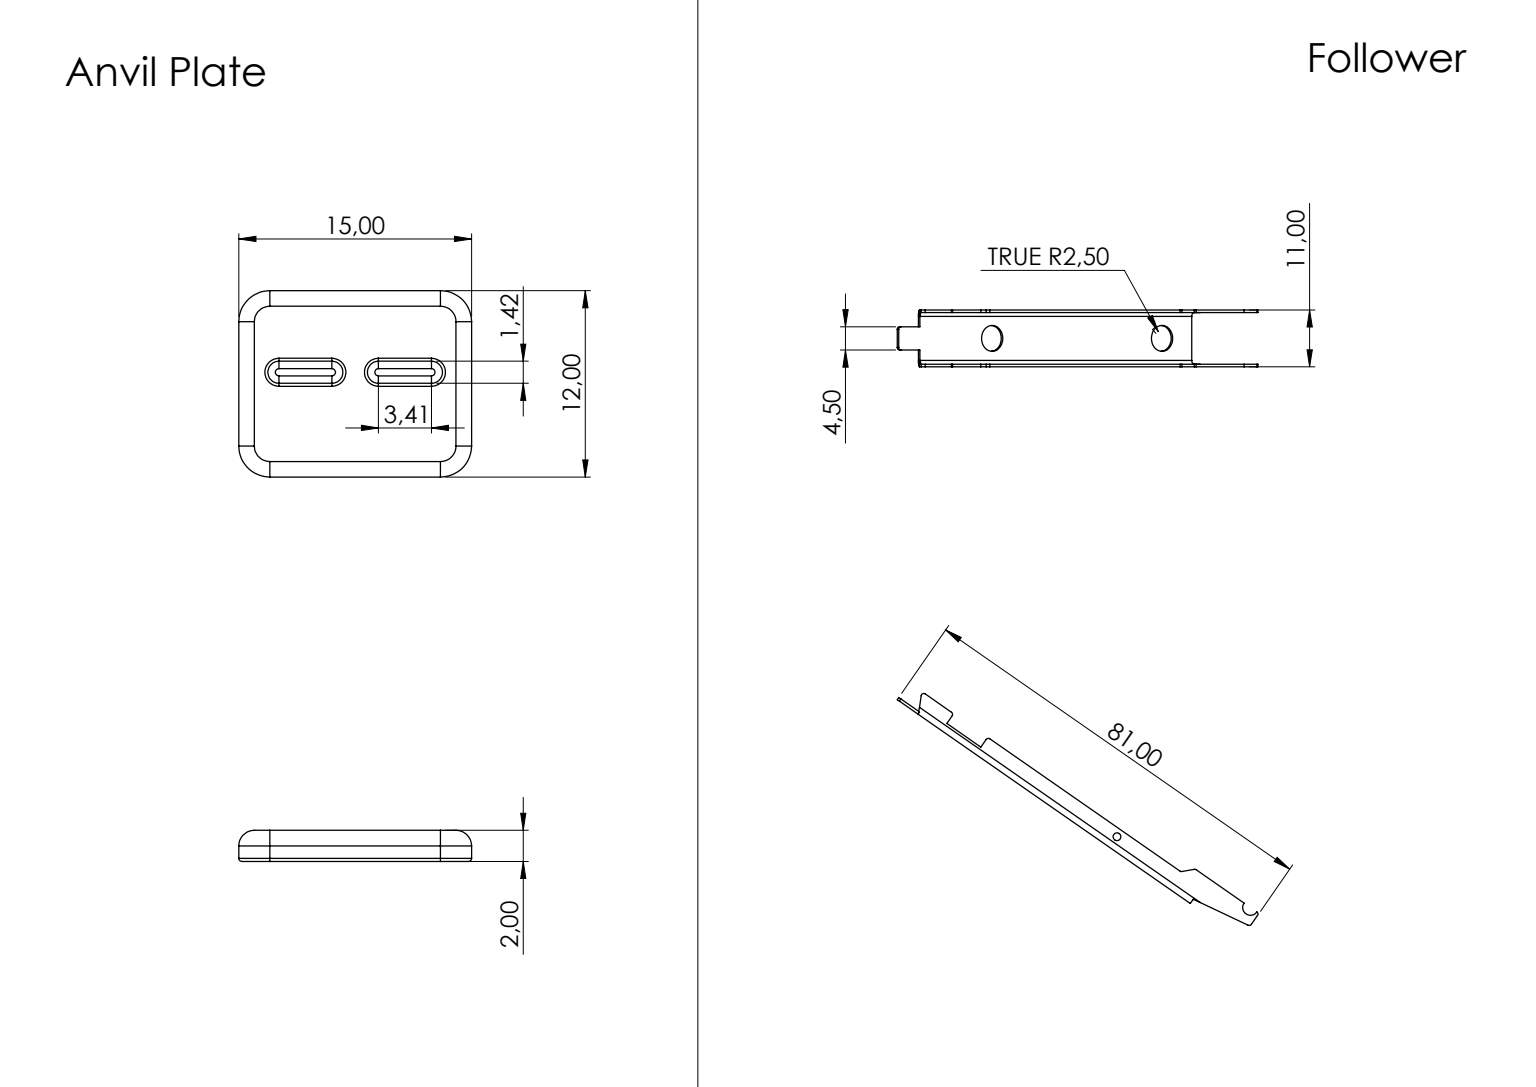
ISO-10303-21;
HEADER;
FILE_DESCRIPTION (('STEP AP214'),
    '1' );
FILE_NAME ('Follower.step',
    '2026-10-06T10:23:46',
    ( '' ),
    ( '' ),
    'SwSTEP 2.0',
    'SolidWorks 2020',
    '' );
FILE_SCHEMA (( 'AUTOMOTIVE_DESIGN' ));
ENDSEC;

DATA;
#8=FACE_OUTER_BOUND ( 'NONE', #24823, .T. ) ;
#39=B_SPLINE_SURFACE_WITH_KNOTS ( 'NONE', 1, 3, ( 
 ( #3682, #6010, #7951, #7688 ),
 ( #11564, #15795, #4076, #7569 ) ),
 .UNSPECIFIED., .F., .F., .F.,
 ( 2, 2 ),
 ( 4, 4 ),
 ( 0.000000000000000000, 1.000000000000000000 ),
 ( 0.000000000000000000, 1.000000000000000000 ),
 .UNSPECIFIED. ) ;
#42=ORIENTED_EDGE ( 'NONE', *, *, #4052, .T. ) ;
#43=CARTESIAN_POINT ( 'NONE',  ( 33.24020206407681144, 3.104049617356281932, 6.135536031321588091 ) ) ;
#48=AXIS2_PLACEMENT_3D ( 'NONE', #18248, #195, #19789 ) ;
#56=ORIENTED_EDGE ( 'NONE', *, *, #3919, .F. ) ;
#59=VERTEX_POINT ( 'NONE', #24601 ) ;
#81=CARTESIAN_POINT ( 'NONE',  ( 43.81606138205700063, -33.39268736607245103, 60.15578379404454523 ) ) ;
#87=VECTOR ( 'NONE', #691, 1000.000000000000114 ) ;
#100=DIRECTION ( 'NONE',  ( 0.000000000000000000, -0.5706330172266907974, 0.8212051873014217795 ) ) ;
#109=EDGE_CURVE ( 'NONE', #2100, #16742, #24351, .T. ) ;
#130=FACE_OUTER_BOUND ( 'NONE', #3742, .T. ) ;
#134=DIRECTION ( 'NONE',  ( 0.000000000000000000, -0.8212051873014223347, -0.5706330172266899092 ) ) ;
#140=CARTESIAN_POINT ( 'NONE',  ( 33.63257508155574271, 2.837830513113388076, 6.099065269017614810 ) ) ;
#156=ORIENTED_EDGE ( 'NONE', *, *, #18156, .F. ) ;
#170=VERTEX_POINT ( 'NONE', #12668 ) ;
#182=CARTESIAN_POINT ( 'NONE',  ( 42.90896497783001706, 3.030042170879425178, 6.235548050178295831 ) ) ;
#195=DIRECTION ( 'NONE',  ( 1.000000000000000000, -0.000000000000000000, 0.000000000000000000 ) ) ;
#198=EDGE_CURVE ( 'NONE', #24709, #13605, #5816, .T. ) ;
#199=EDGE_CURVE ( 'NONE', #8460, #24765, #19336, .T. ) ;
#205=LINE ( 'NONE', #24148, #14945 ) ;
#230=DIRECTION ( 'NONE',  ( 1.000000000000000000, 1.518641380243644581E-16, 1.055262346480601087E-16 ) ) ;
#232=CARTESIAN_POINT ( 'NONE',  ( 32.81606138205700773, -27.11289203277224402, 56.96090842897168471 ) ) ;
#233=DIRECTION ( 'NONE',  ( -1.849283715844614702E-16, 0.8212051873014210024, 0.5706330172266920187 ) ) ;
#252=ADVANCED_FACE ( 'NONE', ( #23316 ), #17669, .F. ) ;
#281=DIRECTION ( 'NONE',  ( 1.000000000000000000, 1.187136597504755470E-16, 8.249087426255173666E-17 ) ) ;
#295=B_SPLINE_CURVE_WITH_KNOTS ( 'NONE', 3,
 ( #12547, #1271, #23035, #14456, #20383, #15309, #9152 ),
 .UNSPECIFIED., .F., .F.,
 ( 4, 3, 4 ),
 ( 0.000000000000000000, 0.9999934796777874002, 1.000000000000000000 ),
 .UNSPECIFIED. ) ;
#300=DIRECTION ( 'NONE',  ( 0.000000000000000000, -0.8212051873014210024, -0.5706330172266920187 ) ) ;
#303=ORIENTED_EDGE ( 'NONE', *, *, #10224, .F. ) ;
#326=CARTESIAN_POINT ( 'NONE',  ( 42.82259893474252266, 3.224890024296139135, 6.370941811568299862 ) ) ;
#340=CARTESIAN_POINT ( 'NONE',  ( 35.81606138205700063, -6.549308025893449070, 20.35783565644092619 ) ) ;
#350=CARTESIAN_POINT ( 'NONE',  ( 42.98956905832248765, 3.335839619497401376, 6.349669990345183201 ) ) ;
#354=DIRECTION ( 'NONE',  ( -0.6683808861234329379, -0.6108281792586462977, -0.4244477900618892630 ) ) ;
#366=VECTOR ( 'NONE', #18918, 1000.000000000000114 ) ;
#374=CYLINDRICAL_SURFACE ( 'NONE', #2185, 1.500000000000006217 ) ;
#377=DIRECTION ( 'NONE',  ( 0.000000000000000000, 0.8212051873014208914, 0.5706330172266919076 ) ) ;
#406=ORIENTED_EDGE ( 'NONE', *, *, #18732, .F. ) ;
#420=ADVANCED_FACE ( 'NONE', ( #130 ), #10070, .F. ) ;
#422=EDGE_CURVE ( 'NONE', #6624, #2302, #15968, .T. ) ;
#435=ORIENTED_EDGE ( 'NONE', *, *, #25058, .T. ) ;
#455=ORIENTED_EDGE ( 'NONE', *, *, #16653, .F. ) ;
#468=EDGE_LOOP ( 'NONE', ( #17209, #1468 ) ) ;
#469=DIRECTION ( 'NONE',  ( 1.444147469618246167E-16, -0.8212051873014210024, -0.5706330172266920187 ) ) ;
#494=ORIENTED_EDGE ( 'NONE', *, *, #8342, .T. ) ;
#513=AXIS2_PLACEMENT_3D ( 'NONE', #8102, #24168, #14160 ) ;
#514=CARTESIAN_POINT ( 'NONE',  ( 33.31606138205700773, -20.26871824316192061, 44.92082169825412308 ) ) ;
#530=EDGE_LOOP ( 'NONE', ( #17922, #3533, #2092, #3855 ) ) ;
#538=PLANE ( 'NONE',  #4659 ) ;
#543=AXIS2_PLACEMENT_3D ( 'NONE', #16608, #5020, #14671 ) ;
#554=EDGE_CURVE ( 'NONE', #25393, #22104, #18436, .T. ) ;
#556=DIRECTION ( 'NONE',  ( 0.000000000000000000, -0.8212051873014223347, -0.5706330172266899092 ) ) ;
#564=CARTESIAN_POINT ( 'NONE',  ( 36.06606138205700063, 3.151453266960317023, 6.397347472316774031 ) ) ;
#592=DIRECTION ( 'NONE',  ( 0.000000000000000000, -0.5706330172266919076, 0.8212051873014208914 ) ) ;
#601=CARTESIAN_POINT ( 'NONE',  ( 32.81606138205700773, 6.705285648480822758, 7.416521610403067122 ) ) ;
#630=CARTESIAN_POINT ( 'NONE',  ( 32.81606138205700773, -35.82531359714782582, 71.25150419970752580 ) ) ;
#633=DIRECTION ( 'NONE',  ( 1.445602896647339656E-16, -0.8212051873014208914, -0.5706330172266919076 ) ) ;
#638=LINE ( 'NONE', #8521, #20462 ) ;
#644=CARTESIAN_POINT ( 'NONE',  ( 33.57054761034910229, 3.412271088041349820, 6.349711998884802533 ) ) ;
#681=ORIENTED_EDGE ( 'NONE', *, *, #198, .T. ) ;
#682=ORIENTED_EDGE ( 'NONE', *, *, #24180, .T. ) ;
#689=ORIENTED_EDGE ( 'NONE', *, *, #21380, .T. ) ;
#691=DIRECTION ( 'NONE',  ( 0.000000000000000000, -0.5706330172266919076, 0.8212051873014208914 ) ) ;
#696=AXIS2_PLACEMENT_3D ( 'NONE', #4403, #12150, #17812 ) ;
#699=EDGE_CURVE ( 'NONE', #20637, #17728, #13096, .T. ) ;
#702=ORIENTED_EDGE ( 'NONE', *, *, #17759, .F. ) ;
#713=CIRCLE ( 'NONE', #8125, 2.500000000000002220 ) ;
#769=VECTOR ( 'NONE', #7198, 1000.000000000000114 ) ;
#788=B_SPLINE_CURVE_WITH_KNOTS ( 'NONE', 3,
 ( #10750, #931, #8822, #10874 ),
 .UNSPECIFIED., .F., .F.,
 ( 4, 4 ),
 ( 0.000000000000000000, 1.000000000000000000 ),
 .UNSPECIFIED. ) ;
#792=CARTESIAN_POINT ( 'NONE',  ( 33.31606138205700773, -27.17722769842920272, 59.42551550655435477 ) ) ;
#794=LINE ( 'NONE', #9887, #17878 ) ;
#798=ORIENTED_EDGE ( 'NONE', *, *, #889, .T. ) ;
#801=DIRECTION ( 'NONE',  ( 1.444147469618246167E-16, -0.8212051873014210024, -0.5706330172266920187 ) ) ;
#814=ORIENTED_EDGE ( 'NONE', *, *, #2858, .T. ) ;
#816=CARTESIAN_POINT ( 'NONE',  ( 42.99361969242278292, 2.839052459004266726, 6.102834979010582472 ) ) ;
#818=VECTOR ( 'NONE', #17657, 1000.000000000000114 ) ;
#833=DIRECTION ( 'NONE',  ( 0.000000000000000000, -0.8212051873014208914, -0.5706330172266919076 ) ) ;
#839=EDGE_CURVE ( 'NONE', #20815, #9471, #19260, .T. ) ;
#853=LINE ( 'NONE', #22510, #16556 ) ;
#855=DIRECTION ( 'NONE',  ( 1.000000000000000000, -0.000000000000000000, 0.000000000000000000 ) ) ;
#860=CYLINDRICAL_SURFACE ( 'NONE', #7319, 0.4999999999999998890 ) ;
#861=B_SPLINE_CURVE_WITH_KNOTS ( 'NONE', 3,
 ( #25078, #7720, #7463, #19426 ),
 .UNSPECIFIED., .F., .F.,
 ( 4, 4 ),
 ( 0.000000000000000000, 1.000000000000000000 ),
 .UNSPECIFIED. ) ;
#864=ORIENTED_EDGE ( 'NONE', *, *, #11208, .F. ) ;
#872=DIRECTION ( 'NONE',  ( 1.000000000000000000, -0.000000000000000000, 0.000000000000000000 ) ) ;
#887=AXIS2_PLACEMENT_3D ( 'NONE', #14310, #8262, #20232 ) ;
#889=EDGE_CURVE ( 'NONE', #2214, #17745, #3160, .T. ) ;
#892=CARTESIAN_POINT ( 'NONE',  ( 43.81606138205700063, -27.52349462642295208, 56.67559192035834315 ) ) ;
#897=CARTESIAN_POINT ( 'NONE',  ( 33.31606138205700773, -2.088476903695762665, 19.19551655256602984 ) ) ;
#922=VECTOR ( 'NONE', #13989, 1000.000000000000114 ) ;
#926=DIRECTION ( 'NONE',  ( 0.000000000000000000, 0.8212051873014208914, 0.5706330172266919076 ) ) ;
#931=CARTESIAN_POINT ( 'NONE',  ( 33.56669025312649524, 3.416671603466172602, 6.349359658337577983 ) ) ;
#933=AXIS2_PLACEMENT_3D ( 'NONE', #16052, #8463, #9892 ) ;
#952=VERTEX_POINT ( 'NONE', #19387 ) ;
#960=ORIENTED_EDGE ( 'NONE', *, *, #16869, .T. ) ;
#965=FACE_OUTER_BOUND ( 'NONE', #17968, .T. ) ;
#967=CIRCLE ( 'NONE', #4280, 0.4999999999999994449 ) ;
#998=CARTESIAN_POINT ( 'NONE',  ( 43.06468080341912241, 3.415100481987971115, 6.350457055188933886 ) ) ;
#999=FACE_OUTER_BOUND ( 'NONE', #16254, .T. ) ;
#1002=VERTEX_POINT ( 'NONE', #21585 ) ;
#1004=CARTESIAN_POINT ( 'NONE',  ( 32.81606138205700773, -27.11289203277224402, 56.96090842897168471 ) ) ;
#1005=ORIENTED_EDGE ( 'NONE', *, *, #20302, .F. ) ;
#1025=FACE_OUTER_BOUND ( 'NONE', #16753, .T. ) ;
#1040=EDGE_CURVE ( 'NONE', #24026, #19555, #16326, .T. ) ;
#1042=EDGE_CURVE ( 'NONE', #9104, #4853, #5608, .T. ) ;
#1044=DIRECTION ( 'NONE',  ( 1.000000000000000000, -0.000000000000000000, 0.000000000000000000 ) ) ;
#1067=ORIENTED_EDGE ( 'NONE', *, *, #19250, .F. ) ;
#1068=DIRECTION ( 'NONE',  ( 1.000000000000000000, -0.000000000000000000, 0.000000000000000000 ) ) ;
#1080=LINE ( 'NONE', #15257, #5531 ) ;
#1082=FACE_OUTER_BOUND ( 'NONE', #2152, .T. ) ;
#1090=CARTESIAN_POINT ( 'NONE',  ( 42.56606138205700063, -32.75315594507191008, 59.38245422252773409 ) ) ;
#1100=CARTESIAN_POINT ( 'NONE',  ( 43.39709375099405975, 3.108381023609500193, 6.137326095127844994 ) ) ;
#1101=CARTESIAN_POINT ( 'NONE',  ( 33.31606138205700773, -26.01295748837380373, 65.89261741282676610 ) ) ;
#1103=AXIS2_PLACEMENT_3D ( 'NONE', #24593, #16498, #10723 ) ;
#1120=CIRCLE ( 'NONE', #696, 0.4999999999999982792 ) ;
#1124=EDGE_CURVE ( 'NONE', #13033, #3938, #8531, .T. ) ;
#1136=AXIS2_PLACEMENT_3D ( 'NONE', #5636, #11329, #11196 ) ;
#1146=LINE ( 'NONE', #22672, #19035 ) ;
#1159=CARTESIAN_POINT ( 'NONE',  ( 32.81606138205700773, -20.26871824316192061, 44.92082169825412308 ) ) ;
#1165=CARTESIAN_POINT ( 'NONE',  ( 32.81606138205700773, -3.566646240838321269, 18.16837712155798457 ) ) ;
#1169=ORIENTED_EDGE ( 'NONE', *, *, #18390, .F. ) ;
#1176=DIRECTION ( 'NONE',  ( -1.000000000000000000, 4.152573584826051666E-20, -5.976021130153593973E-20 ) ) ;
#1182=ORIENTED_EDGE ( 'NONE', *, *, #7364, .T. ) ;
#1191=LINE ( 'NONE', #21171, #9841 ) ;
#1194=CARTESIAN_POINT ( 'NONE',  ( 43.81608638205700146, -3.566646240838321269, 18.16837712155798457 ) ) ;
#1200=CARTESIAN_POINT ( 'NONE',  ( 32.81606138205700773, -27.60498114914039647, 57.04949906928990089 ) ) ;
#1203=VECTOR ( 'NONE', #13238, 999.9999999999998863 ) ;
#1207=CARTESIAN_POINT ( 'NONE',  ( 43.24580177837434292, 3.721690752961224202, 6.335617458560805382 ) ) ;
#1212=LINE ( 'NONE', #10894, #2646 ) ;
#1240=DIRECTION ( 'NONE',  ( 1.000000000000000000, -0.000000000000000000, 0.000000000000000000 ) ) ;
#1262=CARTESIAN_POINT ( 'NONE',  ( 33.31606138205700773, 6.366250835946937414, 6.636353555660924997 ) ) ;
#1271=CARTESIAN_POINT ( 'NONE',  ( 42.65336712727322777, 3.163553052512885877, 6.379934517999310550 ) ) ;
#1304=ORIENTED_EDGE ( 'NONE', *, *, #10169, .T. ) ;
#1316=EDGE_CURVE ( 'NONE', #2214, #22818, #6046, .T. ) ;
#1321=DIRECTION ( 'NONE',  ( 0.000000000000000000, 0.5706330172266920187, -0.8212051873014210024 ) ) ;
#1332=CARTESIAN_POINT ( 'NONE',  ( 33.23377616717382921, 3.110315666471061391, 6.136481299340784012 ) ) ;
#1348=CARTESIAN_POINT ( 'NONE',  ( 32.81606138205700773, -1.677874310045055051, 19.48083306117937852 ) ) ;
#1371=AXIS2_PLACEMENT_3D ( 'NONE', #16139, #21574, #22069 ) ;
#1372=ORIENTED_EDGE ( 'NONE', *, *, #7692, .T. ) ;
#1377=ADVANCED_FACE ( 'NONE', ( #1082 ), #8967, .T. ) ;
#1392=CARTESIAN_POINT ( 'NONE',  ( 43.31606138205700063, 6.355893005198818280, 6.643287643123708008 ) ) ;
#1412=LINE ( 'NONE', #8779, #21644 ) ;
#1433=DIRECTION ( 'NONE',  ( -1.000000000000000000, 0.000000000000000000, 0.000000000000000000 ) ) ;
#1447=VECTOR ( 'NONE', #3335, 1000.000000000000114 ) ;
#1449=DIRECTION ( 'NONE',  ( 0.000000000000000000, 0.8212051873014208914, 0.5706330172266919076 ) ) ;
#1459=ORIENTED_EDGE ( 'NONE', *, *, #3158, .F. ) ;
#1467=CARTESIAN_POINT ( 'NONE',  ( 43.70349364522802205, 3.546438648963166962, 6.213839566231161626 ) ) ;
#1468=ORIENTED_EDGE ( 'NONE', *, *, #8169, .T. ) ;
#1472=CARTESIAN_POINT ( 'NONE',  ( 32.81606138205700773, -21.50052602411404834, 44.06487217241408416 ) ) ;
#1477=CARTESIAN_POINT ( 'NONE',  ( 43.81606138205700063, -27.11289203277224402, 56.96090842897168471 ) ) ;
#1480=CARTESIAN_POINT ( 'NONE',  ( 43.79080625344859357, -32.95845724189726411, 59.23979596822106686 ) ) ;
#1491=ADVANCED_FACE ( 'NONE', ( #15640 ), #17326, .F. ) ;
#1495=CARTESIAN_POINT ( 'NONE',  ( 42.56606138205700063, 3.151453266960317023, 6.397347472316774031 ) ) ;
#1509=CARTESIAN_POINT ( 'NONE',  ( 43.38751061443460344, 3.099069811988895751, 6.135932541694130826 ) ) ;
#1510=VERTEX_POINT ( 'NONE', #1472 ) ;
#1523=CARTESIAN_POINT ( 'NONE',  ( 33.71979045277213061, 3.032422752665409060, 6.234282092415138976 ) ) ;
#1525=ADVANCED_FACE ( 'NONE', ( #3920 ), #7918, .F. ) ;
#1526=CARTESIAN_POINT ( 'NONE',  ( 43.79080625344859357, -32.95845724189726411, 59.23979596822106686 ) ) ;
#1537=VERTEX_POINT ( 'NONE', #25024 ) ;
#1543=ORIENTED_EDGE ( 'NONE', *, *, #2231, .T. ) ;
#1547=ORIENTED_EDGE ( 'NONE', *, *, #2650, .T. ) ;
#1559=AXIS2_PLACEMENT_3D ( 'NONE', #18264, #6280, #592 ) ;
#1585=DIRECTION ( 'NONE',  ( 1.000000000000000000, -0.000000000000000000, 0.000000000000000000 ) ) ;
#1588=VECTOR ( 'NONE', #24821, 1000.000000000000000 ) ;
#1595=CIRCLE ( 'NONE', #11502, 0.4999999999999943379 ) ;
#1603=ORIENTED_EDGE ( 'NONE', *, *, #4465, .F. ) ;
#1614=ORIENTED_EDGE ( 'NONE', *, *, #11768, .T. ) ;
#1617=CARTESIAN_POINT ( 'NONE',  ( 42.99670445188912282, 2.835726111602991040, 6.100265081570795722 ) ) ;
#1626=FACE_OUTER_BOUND ( 'NONE', #15605, .T. ) ;
#1628=CARTESIAN_POINT ( 'NONE',  ( 43.81606138205700063, -2.088476903695762665, 19.19551655256602984 ) ) ;
#1643=AXIS2_PLACEMENT_3D ( 'NONE', #20107, #18312, #377 ) ;
#1648=VECTOR ( 'NONE', #872, 1000.000000000000000 ) ;
#1657=LINE ( 'NONE', #23301, #818 ) ;
#1658=VERTEX_POINT ( 'NONE', #2351 ) ;
#1677=LINE ( 'NONE', #21275, #16046 ) ;
#1680=CARTESIAN_POINT ( 'NONE',  ( 33.91846891627784544, 2.749301080711977985, 6.091107676698986673 ) ) ;
#1682=DIRECTION ( 'NONE',  ( 0.000000000000000000, 0.8212051873014208914, 0.5706330172266919076 ) ) ;
#1683=EDGE_CURVE ( 'NONE', #18636, #16606, #16266, .T. ) ;
#1687=DIRECTION ( 'NONE',  ( 0.000000000000000000, 0.5706330172266920187, -0.8212051873014210024 ) ) ;
#1735=ORIENTED_EDGE ( 'NONE', *, *, #22580, .T. ) ;
#1746=ORIENTED_EDGE ( 'NONE', *, *, #21067, .T. ) ;
#1750=DIRECTION ( 'NONE',  ( -1.000000000000000000, -4.949452455753099023E-16, 7.122819585028524934E-16 ) ) ;
#1752=DIRECTION ( 'NONE',  ( 0.000000000000000000, -0.5706330172266907974, 0.8212051873014217795 ) ) ;
#1783=CARTESIAN_POINT ( 'NONE',  ( 35.81606138205700063, -29.78523130861184498, 52.92072663988442116 ) ) ;
#1801=DIRECTION ( 'NONE',  ( -1.000000000000000000, 0.000000000000000000, 0.000000000000000000 ) ) ;
#1816=DIRECTION ( 'NONE',  ( -1.000000000000000000, 0.000000000000000000, 0.000000000000000000 ) ) ;
#1847=ORIENTED_EDGE ( 'NONE', *, *, #19132, .T. ) ;
#1855=CARTESIAN_POINT ( 'NONE',  ( 43.80758610329830560, -33.17626767724734549, 59.69730752409159180 ) ) ;
#1860=ORIENTED_EDGE ( 'NONE', *, *, #12473, .T. ) ;
#1861=CARTESIAN_POINT ( 'NONE',  ( 43.81606138205700063, 6.699978067258562042, 7.424159817622362212 ) ) ;
#1882=DIRECTION ( 'NONE',  ( 0.000000000000000000, -0.5706330172266919076, 0.8212051873014208914 ) ) ;
#1890=ORIENTED_EDGE ( 'NONE', *, *, #8714, .T. ) ;
#1893=ORIENTED_EDGE ( 'NONE', *, *, #12474, .F. ) ;
#1898=CARTESIAN_POINT ( 'NONE',  ( 36.06606138205700063, 5.308699250829721272, 2.416607620847027960 ) ) ;
#1929=VECTOR ( 'NONE', #6753, 1000.000000000000114 ) ;
#1938=CARTESIAN_POINT ( 'NONE',  ( 34.06606138205700773, 2.736744647373095418, 6.109177798617293931 ) ) ;
#1946=AXIS2_PLACEMENT_3D ( 'NONE', #15039, #5257, #19545 ) ;
#1955=CARTESIAN_POINT ( 'NONE',  ( 40.06606138205700063, 5.594015759443068170, 2.006005027196319901 ) ) ;
#1964=AXIS2_PLACEMENT_3D ( 'NONE', #22242, #18267, #23913 ) ;
#1967=SURFACE_STYLE_USAGE ( .BOTH. , #7915 ) ;
#1973=LINE ( 'NONE', #9856, #22899 ) ;
#2000=AXIS2_PLACEMENT_3D ( 'NONE', #9286, #12766, #22537 ) ;
#2007=ORIENTED_EDGE ( 'NONE', *, *, #17291, .T. ) ;
#2021=AXIS2_PLACEMENT_3D ( 'NONE', #13128, #4749, #12753 ) ;
#2025=ORIENTED_EDGE ( 'NONE', *, *, #18387, .T. ) ;
#2026=VERTEX_POINT ( 'NONE', #3621 ) ;
#2039=CARTESIAN_POINT ( 'NONE',  ( 33.31606138205700773, -33.70281195181703993, 69.07320514641659770 ) ) ;
#2053=ORIENTED_EDGE ( 'NONE', *, *, #3718, .F. ) ;
#2060=PLANE ( 'NONE',  #11156 ) ;
#2064=CARTESIAN_POINT ( 'NONE',  ( 40.56606138205700773, 3.151453266960317023, 6.397347472316774031 ) ) ;
#2069=FACE_OUTER_BOUND ( 'NONE', #20298, .T. ) ;
#2070=VECTOR ( 'NONE', #18574, 1000.000000000000000 ) ;
#2092=ORIENTED_EDGE ( 'NONE', *, *, #11384, .F. ) ;
#2100=VERTEX_POINT ( 'NONE', #21035 ) ;
#2110=DIRECTION ( 'NONE',  ( 0.000000000000000000, -0.5706330172266913525, 0.8212051873014213355 ) ) ;
#2118=DIRECTION ( 'NONE',  ( -1.000000000000000000, 0.000000000000000000, 0.000000000000000000 ) ) ;
#2134=VERTEX_POINT ( 'NONE', #17170 ) ;
#2136=DIRECTION ( 'NONE',  ( 0.000000000000000000, -0.5706330172266919076, 0.8212051873014208914 ) ) ;
#2138=LINE ( 'NONE', #18006, #20063 ) ;
#2139=DIRECTION ( 'NONE',  ( -1.000000000000000000, -1.187136597504755470E-16, -8.249087426255173666E-17 ) ) ;
#2151=EDGE_CURVE ( 'NONE', #23532, #22006, #19727, .T. ) ;
#2152=EDGE_LOOP ( 'NONE', ( #3581, #6754, #7192, #10219 ) ) ;
#2157=VECTOR ( 'NONE', #20748, 1000.000000000000000 ) ;
#2163=ADVANCED_FACE ( 'NONE', ( #19632 ), #15390, .F. ) ;
#2166=CARTESIAN_POINT ( 'NONE',  ( 42.99362197529018914, 2.839053354292388143, 6.102835146812753742 ) ) ;
#2168=VECTOR ( 'NONE', #22569, 1000.000000000000114 ) ;
#2174=CARTESIAN_POINT ( 'NONE',  ( 38.31606138205700063, -29.78523130861184143, 52.92072663988442116 ) ) ;
#2185=AXIS2_PLACEMENT_3D ( 'NONE', #8014, #22033, #15852 ) ;
#2193=DIRECTION ( 'NONE',  ( -1.000000000000000000, 0.000000000000000000, 0.000000000000000000 ) ) ;
#2206=B_SPLINE_CURVE_WITH_KNOTS ( 'NONE', 3,
 ( #8105, #15951, #2539, #6429, #4246, #10424 ),
 .UNSPECIFIED., .F., .F.,
 ( 4, 2, 4 ),
 ( 0.000000000000000000, 0.5000000000000000000, 1.000000000000000000 ),
 .UNSPECIFIED. ) ;
#2207=CARTESIAN_POINT ( 'NONE',  ( 43.21596744901363962, 3.650325757544471195, 6.335220020744675828 ) ) ;
#2214=VERTEX_POINT ( 'NONE', #13842 ) ;
#2225=AXIS2_PLACEMENT_3D ( 'NONE', #3016, #16941, #7154 ) ;
#2231=EDGE_CURVE ( 'NONE', #3938, #16606, #1973, .T. ) ;
#2244=DIRECTION ( 'NONE',  ( 0.6571615412467028960, -0.6189832172005511612, -0.4301145028132777881 ) ) ;
#2259=DIRECTION ( 'NONE',  ( -1.000000000000000000, 0.000000000000000000, 0.000000000000000000 ) ) ;
#2267=CARTESIAN_POINT ( 'NONE',  ( 32.81606138205700773, 2.740850673309605412, 6.112030963703427133 ) ) ;
#2271=AXIS2_PLACEMENT_3D ( 'NONE', #630, #4518, #19980 ) ;
#2295=LINE ( 'NONE', #5926, #23610 ) ;
#2302=VERTEX_POINT ( 'NONE', #23240 ) ;
#2322=EDGE_CURVE ( 'NONE', #6643, #22414, #10576, .T. ) ;
#2335=VECTOR ( 'NONE', #4912, 1000.000000000000114 ) ;
#2351=CARTESIAN_POINT ( 'NONE',  ( 43.81606138205700063, 0.9984178969752143251, 11.59873562314662010 ) ) ;
#2353=VERTEX_POINT ( 'NONE', #10618 ) ;
#2355=CARTESIAN_POINT ( 'NONE',  ( 33.63430211860926278, 2.841683824787794688, 6.101742829876990015 ) ) ;
#2369=AXIS2_PLACEMENT_3D ( 'NONE', #14550, #4758, #9023 ) ;
#2375=VECTOR ( 'NONE', #15926, 1000.000000000000000 ) ;
#2377=ORIENTED_EDGE ( 'NONE', *, *, #11194, .F. ) ;
#2387=ORIENTED_EDGE ( 'NONE', *, *, #23881, .F. ) ;
#2389=ORIENTED_EDGE ( 'NONE', *, *, #12473, .F. ) ;
#2402=EDGE_LOOP ( 'NONE', ( #20983, #1543, #25185, #10638 ) ) ;
#2421=LINE ( 'NONE', #8239, #8598 ) ;
#2459=EDGE_LOOP ( 'NONE', ( #2389, #9279, #960, #1890 ) ) ;
#2493=ORIENTED_EDGE ( 'NONE', *, *, #20622, .F. ) ;
#2498=CARTESIAN_POINT ( 'NONE',  ( 43.31606138205700063, 6.699978067258562042, 7.424159817622362212 ) ) ;
#2504=LINE ( 'NONE', #16287, #25087 ) ;
#2505=CARTESIAN_POINT ( 'NONE',  ( 36.06606138205700063, 6.004618353093779781, 2.291321535809666354 ) ) ;
#2507=CARTESIAN_POINT ( 'NONE',  ( 40.06606138205700063, 5.719301844480432884, 2.701924129460374413 ) ) ;
#2519=PLANE ( 'NONE',  #1559 ) ;
#2536=PLANE ( 'NONE',  #20690 ) ;
#2539=CARTESIAN_POINT ( 'NONE',  ( 32.85323118609061055, 3.754743573466610140, 6.231177976620426051 ) ) ;
#2544=ADVANCED_FACE ( 'NONE', ( #13055 ), #14719, .F. ) ;
#2546=ADVANCED_FACE ( 'NONE', ( #14982 ), #22579, .F. ) ;
#2549=CYLINDRICAL_SURFACE ( 'NONE', #13146, 0.7500000000000006661 ) ;
#2562=CARTESIAN_POINT ( 'NONE',  ( 43.31606138205700063, -37.98241563432385703, 69.85268917996594951 ) ) ;
#2580=CARTESIAN_POINT ( 'NONE',  ( 43.31606138205700063, -27.25871422114667553, 59.79942265548595515 ) ) ;
#2584=CARTESIAN_POINT ( 'NONE',  ( 32.81606138205700773, -40.62725863591898445, 68.52362519861142687 ) ) ;
#2585=CIRCLE ( 'NONE', #16172, 0.5000000000000005551 ) ;
#2590=VERTEX_POINT ( 'NONE', #5067 ) ;
#2595=VERTEX_POINT ( 'NONE', #18723 ) ;
#2600=CARTESIAN_POINT ( 'NONE',  ( 43.81608638205700146, 2.761903742731119049, 12.21527246050395377 ) ) ;
#2642=EDGE_LOOP ( 'NONE', ( #4611, #1847, #18235, #21818 ) ) ;
#2643=ORIENTED_EDGE ( 'NONE', *, *, #23871, .T. ) ;
#2646=VECTOR ( 'NONE', #9349, 1000.000000000000114 ) ;
#2650=EDGE_CURVE ( 'NONE', #3066, #7328, #17172, .T. ) ;
#2651=CARTESIAN_POINT ( 'NONE',  ( 43.38751061443460344, 3.099069811988895751, 6.135932541694130826 ) ) ;
#2656=ORIENTED_EDGE ( 'NONE', *, *, #17591, .T. ) ;
#2663=CARTESIAN_POINT ( 'NONE',  ( 43.31606138205700063, -21.31259689655800216, 45.10875082581016926 ) ) ;
#2684=ADVANCED_FACE ( 'NONE', ( #3624 ), #23078, .T. ) ;
#2693=DIRECTION ( 'NONE',  ( -1.000000000000000000, 0.000000000000000000, 0.000000000000000000 ) ) ;
#2712=LINE ( 'NONE', #23729, #19768 ) ;
#2715=CARTESIAN_POINT ( 'NONE',  ( 43.31606138205700063, -20.45664737071796324, 43.87694304485803798 ) ) ;
#2731=CARTESIAN_POINT ( 'NONE',  ( 33.31606138205700773, 2.761903742731119049, 12.21527246050395377 ) ) ;
#2740=ORIENTED_EDGE ( 'NONE', *, *, #17892, .F. ) ;
#2773=ORIENTED_EDGE ( 'NONE', *, *, #21508, .T. ) ;
#2818=CARTESIAN_POINT ( 'NONE',  ( 43.81606138205700063, 6.355893005198818280, 6.643287643123708008 ) ) ;
#2819=DIRECTION ( 'NONE',  ( 0.000000000000000000, 0.5706330172266919076, -0.8212051873014208914 ) ) ;
#2830=PRODUCT_DEFINITION ( 'UNKNOWN', '', #24844, #11069 ) ;
#2849=CYLINDRICAL_SURFACE ( 'NONE', #11187, 0.7500000000000006661 ) ;
#2858=EDGE_CURVE ( 'NONE', #17088, #24765, #1120, .T. ) ;
#2869=ORIENTED_EDGE ( 'NONE', *, *, #8023, .F. ) ;
#2877=CARTESIAN_POINT ( 'NONE',  ( 33.56477571746443544, 3.418883076854447367, 6.349191931652266696 ) ) ;
#2886=EDGE_LOOP ( 'NONE', ( #15201, #16414, #12183, #5550, #21842, #864, #6325, #14118, #303 ) ) ;
#2894=VECTOR ( 'NONE', #4752, 1000.000000000000114 ) ;
#2938=EDGE_CURVE ( 'NONE', #14856, #17225, #638, .T. ) ;
#2942=CARTESIAN_POINT ( 'NONE',  ( 40.81606138205700773, -29.78523130861184143, 52.92072663988442116 ) ) ;
#2951=VECTOR ( 'NONE', #10283, 1000.000000000000000 ) ;
#2961=ORIENTED_EDGE ( 'NONE', *, *, #21508, .F. ) ;
#2989=AXIS2_PLACEMENT_3D ( 'NONE', #7407, #3271, #22854 ) ;
#2994=CARTESIAN_POINT ( 'NONE',  ( 33.31606138205700773, -21.50052602411404834, 44.06487217241408416 ) ) ;
#3016=CARTESIAN_POINT ( 'NONE',  ( 32.81606138205700773, -2.373793412309109563, 19.60611914621674146 ) ) ;
#3017=VECTOR ( 'NONE', #11670, 1000.000000000000114 ) ;
#3018=EDGE_CURVE ( 'NONE', #25424, #11314, #24461, .T. ) ;
#3020=ORIENTED_EDGE ( 'NONE', *, *, #3910, .T. ) ;
#3022=ORIENTED_EDGE ( 'NONE', *, *, #8029, .F. ) ;
#3044=ORIENTED_EDGE ( 'NONE', *, *, #18005, .T. ) ;
#3057=CARTESIAN_POINT ( 'NONE',  ( 32.81606138205700773, -35.70002751211045933, 71.94742330197156832 ) ) ;
#3066=VERTEX_POINT ( 'NONE', #16490 ) ;
#3075=EDGE_CURVE ( 'NONE', #3766, #18371, #14947, .T. ) ;
#3081=EDGE_LOOP ( 'NONE', ( #23010, #5207, #12290, #19264, #406, #13889, #20963, #24163, #19020, #5502, #9015, #15641, #6393, #18770, #23900, #13377, #22253, #814, #10760 ) ) ;
#3090=FACE_BOUND ( 'NONE', #6509, .T. ) ;
#3108=DIRECTION ( 'NONE',  ( 1.849283715844614949E-16, -0.8212051873014210024, -0.5706330172266920187 ) ) ;
#3109=CARTESIAN_POINT ( 'NONE',  ( 33.31606138205700773, -20.88462213363798270, 44.49284693533410717 ) ) ;
#3135=CARTESIAN_POINT ( 'NONE',  ( 33.23698182036294924, 3.107175835156888333, 6.136003935501333828 ) ) ;
#3136=CARTESIAN_POINT ( 'NONE',  ( 32.81606138205700773, -20.88462213363798270, 44.49284693533410717 ) ) ;
#3143=ORIENTED_EDGE ( 'NONE', *, *, #18547, .T. ) ;
#3149=ORIENTED_EDGE ( 'NONE', *, *, #8029, .T. ) ;
#3152=EDGE_LOOP ( 'NONE', ( #22051, #19916, #9029, #12464 ) ) ;
#3158=EDGE_CURVE ( 'NONE', #25244, #17225, #11738, .T. ) ;
#3160=LINE ( 'NONE', #24791, #12696 ) ;
#3175=CARTESIAN_POINT ( 'NONE',  ( 32.81606138205700773, 2.476587234117772596, 12.62587505415466538 ) ) ;
#3180=CARTESIAN_POINT ( 'NONE',  ( 32.81606138205700773, -26.01295748837380373, 65.89261741282676610 ) ) ;
#3187=FACE_OUTER_BOUND ( 'NONE', #3152, .T. ) ;
#3203=DIRECTION ( 'NONE',  ( -1.000000000000000000, 0.000000000000000000, 0.000000000000000000 ) ) ;
#3218=ORIENTED_EDGE ( 'NONE', *, *, #8621, .T. ) ;
#3234=CARTESIAN_POINT ( 'NONE',  ( 34.06606138205700773, -36.11063010576116739, 71.66210679335823386 ) ) ;
#3238=CARTESIAN_POINT ( 'NONE',  ( 33.56477571746443544, 3.418883076854447367, 6.349191931652266696 ) ) ;
#3249=AXIS2_PLACEMENT_3D ( 'NONE', #2174, #233, #17915 ) ;
#3253=DIRECTION ( 'NONE',  ( 0.000000000000000000, 0.8212051873014210024, 0.5706330172266920187 ) ) ;
#3271=DIRECTION ( 'NONE',  ( 1.000000000000000000, -0.000000000000000000, 0.000000000000000000 ) ) ;
#3278=FILL_AREA_STYLE_COLOUR ( '', #16218 ) ;
#3280=ORIENTED_EDGE ( 'NONE', *, *, #9413, .T. ) ;
#3296=VERTEX_POINT ( 'NONE', #1526 ) ;
#3299=ORIENTED_EDGE ( 'NONE', *, *, #16653, .T. ) ;
#3310=CARTESIAN_POINT ( 'NONE',  ( 42.99807726499842175, 2.836257474661138644, 6.100376100592989737 ) ) ;
#3335=DIRECTION ( 'NONE',  ( -1.849283715844614456E-16, 0.8212051873014208914, 0.5706330172266919076 ) ) ;
#3338=ORIENTED_EDGE ( 'NONE', *, *, #21854, .F. ) ;
#3352=DIRECTION ( 'NONE',  ( 0.000000000000000000, -0.8212051873014252212, -0.5706330172266858014 ) ) ;
#3392=EDGE_LOOP ( 'NONE', ( #19337, #18765, #10376, #22222 ) ) ;
#3396=DIRECTION ( 'NONE',  ( 0.000000000000000000, 0.5706330172266920187, -0.8212051873014210024 ) ) ;
#3410=DIRECTION ( 'NONE',  ( -1.000000000000000000, 0.000000000000000000, 0.000000000000000000 ) ) ;
#3412=EDGE_CURVE ( 'NONE', #17256, #9754, #23558, .T. ) ;
#3419=ORIENTED_EDGE ( 'NONE', *, *, #18856, .T. ) ;
#3421=EDGE_CURVE ( 'NONE', #16162, #19839, #2421, .T. ) ;
#3432=CARTESIAN_POINT ( 'NONE',  ( 43.62725655850141493, 3.386289273678555922, 6.178516409519463792 ) ) ;
#3435=VERTEX_POINT ( 'NONE', #19960 ) ;
#3445=EDGE_CURVE ( 'NONE', #7878, #14092, #9043, .T. ) ;
#3447=CARTESIAN_POINT ( 'NONE',  ( 43.06468080341933558, 3.415100481988189607, 6.350457055188961419 ) ) ;
#3461=ADVANCED_FACE ( 'NONE', ( #8369 ), #19830, .T. ) ;
#3519=CARTESIAN_POINT ( 'NONE',  ( 43.31606138205700063, -3.566646240838321269, 18.16837712155798457 ) ) ;
#3530=B_SPLINE_SURFACE_WITH_KNOTS ( 'NONE', 1, 3, ( 
 ( #1467, #18868, #7017, #17192 ),
 ( #14865, #25018, #11283, #22727 ),
 ( #1207, #9095, #16937, #13078 ) ),
 .UNSPECIFIED., .F., .F., .F.,
 ( 2, 1, 2 ),
 ( 4, 4 ),
 ( -0.01000000000000000021, 0.000000000000000000, 1.000000000000000000 ),
 ( 0.000000000000000000, 1.000000000000000000 ),
 .UNSPECIFIED. ) ;
#3533=ORIENTED_EDGE ( 'NONE', *, *, #9274, .T. ) ;
#3547=ORIENTED_EDGE ( 'NONE', *, *, #9413, .F. ) ;
#3557=CARTESIAN_POINT ( 'NONE',  ( 42.82505858241695762, 3.225987868298963779, 6.370930886792723236 ) ) ;
#3558=ADVANCED_FACE ( 'NONE', ( #3187 ), #12004, .T. ) ;
#3566=CARTESIAN_POINT ( 'NONE',  ( 38.31606138205700063, -6.549308025893449070, 20.35783565644092619 ) ) ;
#3578=EDGE_CURVE ( 'NONE', #19784, #11454, #16590, .T. ) ;
#3581=ORIENTED_EDGE ( 'NONE', *, *, #5626, .F. ) ;
#3600=LINE ( 'NONE', #17021, #21788 ) ;
#3606=VECTOR ( 'NONE', #12428, 1000.000000000000114 ) ;
#3620=CARTESIAN_POINT ( 'NONE',  ( 33.63430211860953278, 2.841683824787687218, 6.101742829876973140 ) ) ;
#3621=CARTESIAN_POINT ( 'NONE',  ( 35.81606138205700063, -29.37462871496113337, 53.20604314849776983 ) ) ;
#3624=FACE_OUTER_BOUND ( 'NONE', #19296, .T. ) ;
#3628=CARTESIAN_POINT ( 'NONE',  ( 32.99554091088187135, 3.410282305729716246, 6.167518378462418127 ) ) ;
#3637=DIRECTION ( 'NONE',  ( 0.000000000000000000, -0.5706330172266913525, 0.8212051873014213355 ) ) ;
#3653=AXIS2_PLACEMENT_3D ( 'NONE', #3699, #25328, #23149 ) ;
#3655=EDGE_CURVE ( 'NONE', #2353, #17597, #11195, .T. ) ;
#3659=SURFACE_STYLE_USAGE ( .BOTH. , #23242 ) ;
#3661=AXIS2_PLACEMENT_3D ( 'NONE', #24456, #19067, #6828 ) ;
#3675=VECTOR ( 'NONE', #21739, 1000.000000000000000 ) ;
#3681=CARTESIAN_POINT ( 'NONE',  ( 36.56606138205700063, 5.308699250829721272, 2.416607620847027960 ) ) ;
#3682=CARTESIAN_POINT ( 'NONE',  ( 32.84131651066541480, -32.95845724189726411, 59.23979596822106686 ) ) ;
#3697=CARTESIAN_POINT ( 'NONE',  ( 33.31606138205700773, -40.62725863591898445, 68.52362519861142687 ) ) ;
#3699=CARTESIAN_POINT ( 'NONE',  ( 43.81606138205700063, -20.88462213363798270, 44.49284693533410717 ) ) ;
#3718=EDGE_CURVE ( 'NONE', #14544, #24541, #22999, .T. ) ;
#3728=EDGE_LOOP ( 'NONE', ( #3768, #15281, #4821, #15902 ) ) ;
#3736=B_SPLINE_SURFACE_WITH_KNOTS ( 'NONE', 1, 3, ( 
 ( #5509, #5756, #19158, #11700, #1617, #3310, #5628 ),
 ( #7310, #13374, #25179, #15161, #11186, #13489, #21221 ),
 ( #1495, #7823, #17231, #15669, #19539, #19034, #3557 ) ),
 .UNSPECIFIED., .F., .F., .F.,
 ( 2, 1, 2 ),
 ( 4, 3, 4 ),
 ( -0.01000000000000000021, 0.000000000000000000, 1.000000000000000000 ),
 ( 0.000000000000000000, 1.000000000000000000, 1.010000000000000009 ),
 .UNSPECIFIED. ) ;
#3741=CARTESIAN_POINT ( 'NONE',  ( 43.81606138205700063, 6.699978067258562042, 7.424159817622362212 ) ) ;
#3742=EDGE_LOOP ( 'NONE', ( #3280, #18043, #11656, #21146 ) ) ;
#3750=DIRECTION ( 'NONE',  ( 0.000000000000000000, -0.5706330172266919076, 0.8212051873014208914 ) ) ;
#3758=DIRECTION ( 'NONE',  ( 0.000000000000000000, -0.8212051873014208914, -0.5706330172266919076 ) ) ;
#3766=VERTEX_POINT ( 'NONE', #23785 ) ;
#3768=ORIENTED_EDGE ( 'NONE', *, *, #18547, .F. ) ;
#3786=CARTESIAN_POINT ( 'NONE',  ( 33.80700705136447937, 3.227014435054107455, 6.369498925975481285 ) ) ;
#3794=CARTESIAN_POINT ( 'NONE',  ( 43.81608638205700146, -3.566646240838321269, 18.16837712155798457 ) ) ;
#3796=ORIENTED_EDGE ( 'NONE', *, *, #23732, .T. ) ;
#3827=CARTESIAN_POINT ( 'NONE',  ( 43.79080625344859357, -32.95845724189726411, 59.23979596822106686 ) ) ;
#3847=CIRCLE ( 'NONE', #13730, 0.7499999999999983347 ) ;
#3852=LINE ( 'NONE', #13276, #21098 ) ;
#3855=ORIENTED_EDGE ( 'NONE', *, *, #20566, .F. ) ;
#3867=ORIENTED_EDGE ( 'NONE', *, *, #11453, .F. ) ;
#3878=CARTESIAN_POINT ( 'NONE',  ( 43.81606138205700063, -37.34243788671330577, 70.80615726751818784 ) ) ;
#3880=DIRECTION ( 'NONE',  ( 1.445602896647339656E-16, -0.8212051873014208914, -0.5706330172266919076 ) ) ;
#3884=LINE ( 'NONE', #19594, #15639 ) ;
#3894=CARTESIAN_POINT ( 'NONE',  ( 43.19824457581059107, 3.616009060170059630, 6.335949910530210616 ) ) ;
#3910=EDGE_CURVE ( 'NONE', #2302, #13705, #25036, .T. ) ;
#3912=ORIENTED_EDGE ( 'NONE', *, *, #2151, .F. ) ;
#3919=EDGE_CURVE ( 'NONE', #9104, #20720, #19566, .T. ) ;
#3920=FACE_OUTER_BOUND ( 'NONE', #13367, .T. ) ;
#3924=ORIENTED_EDGE ( 'NONE', *, *, #22580, .F. ) ;
#3928=PRESENTATION_STYLE_ASSIGNMENT (( #3659 ) ) ;
#3938=VERTEX_POINT ( 'NONE', #9296 ) ;
#3943=ORIENTED_EDGE ( 'NONE', *, *, #17763, .F. ) ;
#3960=EDGE_CURVE ( 'NONE', #19561, #7627, #19191, .T. ) ;
#3965=DIRECTION ( 'NONE',  ( -1.734723475976804876E-16, 0.8212051873014210024, 0.5706330172266920187 ) ) ;
#3967=CARTESIAN_POINT ( 'NONE',  ( 43.39072112803988546, 3.102161780314388828, 6.136388117020111999 ) ) ;
#3990=ORIENTED_EDGE ( 'NONE', *, *, #3421, .F. ) ;
#4018=CARTESIAN_POINT ( 'NONE',  ( 43.16142150209545747, 3.549114036551906270, 6.338043885949037559 ) ) ;
#4036=DIRECTION ( 'NONE',  ( 0.000000000000000000, -0.9911113317706403691, -0.1330350631819583740 ) ) ;
#4037=ORIENTED_EDGE ( 'NONE', *, *, #6413, .F. ) ;
#4040=( LENGTH_UNIT ( ) NAMED_UNIT ( * ) SI_UNIT ( .MILLI., .METRE. ) );
#4051=CARTESIAN_POINT ( 'NONE',  ( 43.81606138205700063, -27.25871422114667553, 59.79942265548595515 ) ) ;
#4052=EDGE_CURVE ( 'NONE', #17088, #2595, #15027, .T. ) ;
#4054=EDGE_CURVE ( 'NONE', #10887, #11457, #17099, .T. ) ;
#4056=CARTESIAN_POINT ( 'NONE',  ( 43.05893433410182070, 3.408565912792066221, 6.350990188909392486 ) ) ;
#4068=CARTESIAN_POINT ( 'NONE',  ( 38.31606138205700063, -29.78523130861184143, 52.92072663988442116 ) ) ;
#4069=UNCERTAINTY_MEASURE_WITH_UNIT (LENGTH_MEASURE( 1.000000000000000082E-05 ), #4040, 'distance_accuracy_value', 'NONE');
#4076=CARTESIAN_POINT ( 'NONE',  ( 33.31606138205700773, -33.36512788127014772, 60.17493381834623989 ) ) ;
#4083=DIRECTION ( 'NONE',  ( -1.849283715844614702E-16, 0.8212051873014210024, 0.5706330172266920187 ) ) ;
#4087=VERTEX_POINT ( 'NONE', #7178 ) ;
#4094=DIRECTION ( 'NONE',  ( 0.000000000000000000, -0.5706330172266952383, 0.8212051873014186709 ) ) ;
#4117=DIRECTION ( 'NONE',  ( 1.849283715844614702E-16, -0.8212051873014210024, -0.5706330172266920187 ) ) ;
#4123=DIRECTION ( 'NONE',  ( 0.000000000000000000, 0.8212051873014210024, 0.5706330172266920187 ) ) ;
#4164=ORIENTED_EDGE ( 'NONE', *, *, #21878, .T. ) ;
#4175=DIRECTION ( 'NONE',  ( -1.000000000000000000, 0.000000000000000000, 0.000000000000000000 ) ) ;
#4204=VECTOR ( 'NONE', #22571, 1000.000000000000000 ) ;
#4209=VECTOR ( 'NONE', #2819, 1000.000000000000114 ) ;
#4222=LINE ( 'NONE', #19936, #3675 ) ;
#4227=VERTEX_POINT ( 'NONE', #564 ) ;
#4240=ORIENTED_EDGE ( 'NONE', *, *, #16024, .F. ) ;
#4246=CARTESIAN_POINT ( 'NONE',  ( 33.10060807238558311, 3.250547983414590281, 6.144371924394154583 ) ) ;
#4249=CARTESIAN_POINT ( 'NONE',  ( 43.31606138205700063, 4.059789041072993321, 6.339735157755647776 ) ) ;
#4251=VECTOR ( 'NONE', #22613, 1000.000000000000114 ) ;
#4258=VECTOR ( 'NONE', #25137, 1000.000000000000227 ) ;
#4271=FACE_OUTER_BOUND ( 'NONE', #20744, .T. ) ;
#4280=AXIS2_PLACEMENT_3D ( 'NONE', #13518, #16547, #4591 ) ;
#4286=EDGE_CURVE ( 'NONE', #10132, #16259, #11121, .T. ) ;
#4305=VECTOR ( 'NONE', #6606, 1000.000000000000227 ) ;
#4308=DIRECTION ( 'NONE',  ( 0.000000000000000000, -0.8212051873014203363, -0.5706330172266926848 ) ) ;
#4344=ORIENTED_EDGE ( 'NONE', *, *, #7602, .T. ) ;
#4345=VERTEX_POINT ( 'NONE', #14733 ) ;
#4358=LINE ( 'NONE', #14020, #25155 ) ;
#4360=VERTEX_POINT ( 'NONE', #11005 ) ;
#4366=CARTESIAN_POINT ( 'NONE',  ( 43.39079911632101272, 3.095977362302465785, 6.133782536096640037 ) ) ;
#4376=ADVANCED_FACE ( 'NONE', ( #24762 ), #17325, .T. ) ;
#4387=EDGE_CURVE ( 'NONE', #3296, #5392, #4927, .T. ) ;
#4395=FACE_OUTER_BOUND ( 'NONE', #5321, .T. ) ;
#4403=CARTESIAN_POINT ( 'NONE',  ( 33.31606138205700773, -27.66931681479738003, 59.51410614687260647 ) ) ;
#4405=CARTESIAN_POINT ( 'NONE',  ( 43.14050698234171222, 3.517279818248786327, 6.340193568624436615 ) ) ;
#4415=ORIENTED_EDGE ( 'NONE', *, *, #9517, .T. ) ;
#4445=DIRECTION ( 'NONE',  ( -1.849283715844614456E-16, 0.8212051873014208914, 0.5706330172266919076 ) ) ;
#4447=VERTEX_POINT ( 'NONE', #1200 ) ;
#4458=CARTESIAN_POINT ( 'NONE',  ( 40.81606138205700773, -6.959910619544160681, 20.07251914782758107 ) ) ;
#4465=EDGE_CURVE ( 'NONE', #22481, #5726, #11933, .T. ) ;
#4494=CARTESIAN_POINT ( 'NONE',  ( 32.81606138205700773, -39.60075215179220720, 69.23691647014479145 ) ) ;
#4511=DIRECTION ( 'NONE',  ( 0.000000000000000000, -0.5706330172266920187, 0.8212051873014210024 ) ) ;
#4518=DIRECTION ( 'NONE',  ( 1.000000000000000000, -0.000000000000000000, 0.000000000000000000 ) ) ;
#4521=EDGE_CURVE ( 'NONE', #1537, #7878, #17314, .T. ) ;
#4543=B_SPLINE_CURVE_WITH_KNOTS ( 'NONE', 3,
 ( #1509, #3967, #5641, #15817 ),
 .UNSPECIFIED., .F., .F.,
 ( 4, 4 ),
 ( 0.000000000000000000, 1.000000000000000000 ),
 .UNSPECIFIED. ) ;
#4551=VERTEX_POINT ( 'NONE', #1955 ) ;
#4561=DIRECTION ( 'NONE',  ( 0.9797958971132711969, -0.1642410374602840950, -0.1141266034453383288 ) ) ;
#4591=DIRECTION ( 'NONE',  ( 0.000000000000000000, -0.5706330172266930179, 0.8212051873014202252 ) ) ;
#4607=VERTEX_POINT ( 'NONE', #21425 ) ;
#4611=ORIENTED_EDGE ( 'NONE', *, *, #21436, .F. ) ;
#4629=VECTOR ( 'NONE', #12230, 1000.000000000000114 ) ;
#4637=AXIS2_PLACEMENT_3D ( 'NONE', #1477, #13352, #21198 ) ;
#4654=CIRCLE ( 'NONE', #14949, 1.250000000000001110 ) ;
#4659=AXIS2_PLACEMENT_3D ( 'NONE', #22191, #17962, #281 ) ;
#4685=CARTESIAN_POINT ( 'NONE',  ( 43.81606138205700063, -34.55876147765707174, 70.30501292736873609 ) ) ;
#4718=CARTESIAN_POINT ( 'NONE',  ( 33.31606138205700773, -37.53049398575952722, 70.06662099985001646 ) ) ;
#4745=DIRECTION ( 'NONE',  ( 1.000000000000000000, -1.144790849096772152E-30, 1.647482979906198098E-30 ) ) ;
#4748=CARTESIAN_POINT ( 'NONE',  ( 43.70349364522802205, 3.546438648963166962, 6.213839566231161626 ) ) ;
#4749=DIRECTION ( 'NONE',  ( 0.000000000000000000, 0.8212051873014210024, 0.5706330172266920187 ) ) ;
#4752=DIRECTION ( 'NONE',  ( 0.000000000000000000, 0.5706330172266919076, -0.8212051873014208914 ) ) ;
#4757=CARTESIAN_POINT ( 'NONE',  ( 42.56606138205700063, -33.77966242919868733, 58.66916295099436951 ) ) ;
#4758=DIRECTION ( 'NONE',  ( -1.000000000000000000, 0.000000000000000000, 0.000000000000000000 ) ) ;
#4770=CARTESIAN_POINT ( 'NONE',  ( 43.31606138205700063, -33.60910547091194900, 60.61426200347987248 ) ) ;
#4776=ORIENTED_EDGE ( 'NONE', *, *, #7275, .T. ) ;
#4795=CARTESIAN_POINT ( 'NONE',  ( 32.81606138205700773, -33.39268736607245103, 60.15578379404453813 ) ) ;
#4799=ORIENTED_EDGE ( 'NONE', *, *, #21380, .F. ) ;
#4821=ORIENTED_EDGE ( 'NONE', *, *, #3421, .T. ) ;
#4822=ORIENTED_EDGE ( 'NONE', *, *, #3960, .F. ) ;
#4824=DIRECTION ( 'NONE',  ( -1.000000000000000000, -1.208430656372714685E-15, -2.875977885193763990E-16 ) ) ;
#4825=ORIENTED_EDGE ( 'NONE', *, *, #16116, .F. ) ;
#4833=EDGE_CURVE ( 'NONE', #19940, #10213, #2712, .T. ) ;
#4845=AXIS2_PLACEMENT_3D ( 'NONE', #10443, #8126, #9940 ) ;
#4853=VERTEX_POINT ( 'NONE', #1165 ) ;
#4886=VECTOR ( 'NONE', #13403, 1000.000000000000000 ) ;
#4893=AXIS2_PLACEMENT_3D ( 'NONE', #3566, #3965, #25459 ) ;
#4912=DIRECTION ( 'NONE',  ( 0.000000000000000000, 0.5706330172266919076, -0.8212051873014208914 ) ) ;
#4927=CIRCLE ( 'NONE', #6166, 1.250000000000001110 ) ;
#4934=AXIS2_PLACEMENT_3D ( 'NONE', #19904, #8437, #556 ) ;
#4964=EDGE_CURVE ( 'NONE', #18040, #13983, #22436, .T. ) ;
#4994=EDGE_CURVE ( 'NONE', #8119, #9175, #19091, .T. ) ;
#5001=LINE ( 'NONE', #12869, #11874 ) ;
#5009=ORIENTED_EDGE ( 'NONE', *, *, #2322, .T. ) ;
#5020=DIRECTION ( 'NONE',  ( 1.000000000000000000, -0.000000000000000000, 0.000000000000000000 ) ) ;
#5041=VECTOR ( 'NONE', #16680, 1000.000000000000000 ) ;
#5055=ORIENTED_EDGE ( 'NONE', *, *, #16869, .F. ) ;
#5057=DIRECTION ( 'NONE',  ( 0.000000000000000000, 0.5706330172266920187, -0.8212051873014210024 ) ) ;
#5067=CARTESIAN_POINT ( 'NONE',  ( 43.81606138205700063, 2.476587234117772596, 12.62587505415466538 ) ) ;
#5082=ORIENTED_EDGE ( 'NONE', *, *, #9738, .T. ) ;
#5083=CARTESIAN_POINT ( 'NONE',  ( 33.24020206407681144, 3.104049617356285040, 6.135536031321588091 ) ) ;
#5090=CARTESIAN_POINT ( 'NONE',  ( 43.69896204258590444, 3.548173818309678484, 6.215045287937394747 ) ) ;
#5099=ORIENTED_EDGE ( 'NONE', *, *, #20649, .F. ) ;
#5137=DIRECTION ( 'NONE',  ( 1.000000000000000000, 0.000000000000000000, 0.000000000000000000 ) ) ;
#5161=LINE ( 'NONE', #4770, #2157 ) ;
#5172=ORIENTED_EDGE ( 'NONE', *, *, #422, .F. ) ;
#5174=ADVANCED_FACE ( 'NONE', ( #9314 ), #23063, .F. ) ;
#5187=PLANE ( 'NONE',  #9272 ) ;
#5191=CARTESIAN_POINT ( 'NONE',  ( 34.06606138205700773, -39.60075215179220720, 69.23691647014479145 ) ) ;
#5196=CARTESIAN_POINT ( 'NONE',  ( 32.81606138205700773, -27.66931681479738003, 59.51410614687260647 ) ) ;
#5207=ORIENTED_EDGE ( 'NONE', *, *, #25128, .T. ) ;
#5208=VERTEX_POINT ( 'NONE', #24192 ) ;
#5214=ORIENTED_EDGE ( 'NONE', *, *, #6903, .T. ) ;
#5229=EDGE_LOOP ( 'NONE', ( #23204, #15684, #19840, #7719 ) ) ;
#5243=CIRCLE ( 'NONE', #8535, 2.500000000000002220 ) ;
#5257=DIRECTION ( 'NONE',  ( 1.000000000000000000, -0.000000000000000000, 0.000000000000000000 ) ) ;
#5266=CARTESIAN_POINT ( 'NONE',  ( 38.31606138205700063, -6.959910619544160681, 20.07251914782758107 ) ) ;
#5278=ORIENTED_EDGE ( 'NONE', *, *, #3075, .F. ) ;
#5304=ADVANCED_FACE ( 'NONE', ( #10442 ), #2060, .F. ) ;
#5315=FACE_OUTER_BOUND ( 'NONE', #16277, .T. ) ;
#5321=EDGE_LOOP ( 'NONE', ( #23620, #9382, #22718, #15805, #16767, #22196, #23791, #15435 ) ) ;
#5326=CARTESIAN_POINT ( 'NONE',  ( 32.81606138205700773, 4.124002793203064066, 6.312068993173404863 ) ) ;
#5336=ORIENTED_EDGE ( 'NONE', *, *, #20098, .F. ) ;
#5344=CARTESIAN_POINT ( 'NONE',  ( 43.81606138205700063, 4.103895195095678794, 6.341006091748962348 ) ) ;
#5358=CARTESIAN_POINT ( 'NONE',  ( 43.30090830489194786, -32.87633672316712108, 59.29685926994373091 ) ) ;
#5369=EDGE_LOOP ( 'NONE', ( #5055, #12894, #7801, #16896, #7175, #25019, #6610, #5586, #22075, #7490, #4164, #1547, #3299, #13979, #20269, #15713, #6161, #7815, #3020 ) ) ;
#5380=AXIS2_PLACEMENT_3D ( 'NONE', #1004, #6816, #20468 ) ;
#5390=B_SPLINE_SURFACE_WITH_KNOTS ( 'NONE', 1, 3, ( 
 ( #23018, #15542, #19409, #7314 ),
 ( #11575, #9267, #13381, #3447 ) ),
 .UNSPECIFIED., .F., .F., .F.,
 ( 2, 2 ),
 ( 4, 4 ),
 ( 0.000000000000000000, 1.000000000000000000 ),
 ( 0.000000000000000000, 1.000000000000000000 ),
 .UNSPECIFIED. ) ;
#5392=VERTEX_POINT ( 'NONE', #4757 ) ;
#5394=DIRECTION ( 'NONE',  ( -1.000000000000000000, 0.000000000000000000, 0.000000000000000000 ) ) ;
#5400=EDGE_CURVE ( 'NONE', #25120, #22481, #24564, .T. ) ;
#5414=CIRCLE ( 'NONE', #887, 1.500000000000006217 ) ;
#5418=EDGE_LOOP ( 'NONE', ( #7672, #23825, #21806, #9250 ) ) ;
#5421=ORIENTED_EDGE ( 'NONE', *, *, #16024, .T. ) ;
#5428=CARTESIAN_POINT ( 'NONE',  ( 38.31606138205700063, -6.959910619544160681, 20.07251914782758107 ) ) ;
#5433=CARTESIAN_POINT ( 'NONE',  ( 34.06606138205700773, -37.81581049437288300, 70.47722359350072452 ) ) ;
#5446=VECTOR ( 'NONE', #2139, 1000.000000000000000 ) ;
#5447=CARTESIAN_POINT ( 'NONE',  ( 32.81606138205700773, 2.740850673309605412, 6.112030963703427133 ) ) ;
#5458=ORIENTED_EDGE ( 'NONE', *, *, #21854, .T. ) ;
#5470=PLANE ( 'NONE',  #13757 ) ;
#5483=CARTESIAN_POINT ( 'NONE',  ( 43.31606138205700063, -33.36512800456291217, 60.17493404035838012 ) ) ;
#5502=ORIENTED_EDGE ( 'NONE', *, *, #12367, .T. ) ;
#5509=CARTESIAN_POINT ( 'NONE',  ( 42.56606138205700063, 2.736744647373098971, 6.109177798617293931 ) ) ;
#5520=LINE ( 'NONE', #3697, #15964 ) ;
#5531=VECTOR ( 'NONE', #6893, 1000.000000000000114 ) ;
#5536=CARTESIAN_POINT ( 'NONE',  ( 32.81606138205700773, -37.98241563432386414, 69.85268917996594951 ) ) ;
#5550=ORIENTED_EDGE ( 'NONE', *, *, #12112, .F. ) ;
#5566=CARTESIAN_POINT ( 'NONE',  ( 32.81606138205700773, -1.963190818658398173, 19.89143565483009013 ) ) ;
#5586=ORIENTED_EDGE ( 'NONE', *, *, #10169, .F. ) ;
#5608=LINE ( 'NONE', #3794, #9351 ) ;
#5626=EDGE_CURVE ( 'NONE', #18958, #11492, #9510, .T. ) ;
#5628=CARTESIAN_POINT ( 'NONE',  ( 42.99945007810772069, 2.836788837719289802, 6.100487119615180198 ) ) ;
#5636=CARTESIAN_POINT ( 'NONE',  ( 38.31606138205700063, -6.959910619544160681, 20.07251914782758107 ) ) ;
#5641=CARTESIAN_POINT ( 'NONE',  ( 43.39391466435952793, 3.105264735555241629, 6.136852473770347594 ) ) ;
#5648=EDGE_CURVE ( 'NONE', #5726, #11314, #25435, .T. ) ;
#5673=AXIS2_PLACEMENT_3D ( 'NONE', #24775, #15006, #16810 ) ;
#5697=CARTESIAN_POINT ( 'NONE',  ( 33.48677699869404023, 3.517612739349352591, 6.329933951274631099 ) ) ;
#5709=VERTEX_POINT ( 'NONE', #10130 ) ;
#5718=LINE ( 'NONE', #19500, #13714 ) ;
#5726=VERTEX_POINT ( 'NONE', #18245 ) ;
#5748=EDGE_LOOP ( 'NONE', ( #7015, #15333, #13534, #9275 ) ) ;
#5756=CARTESIAN_POINT ( 'NONE',  ( 42.71215467885433270, 2.748844572886082638, 6.091764642881028813 ) ) ;
#5767=EDGE_CURVE ( 'NONE', #18636, #23179, #2504, .T. ) ;
#5769=CARTESIAN_POINT ( 'NONE',  ( 32.81606138205700773, -26.01295748837380373, 65.89261741282676610 ) ) ;
#5793=EDGE_CURVE ( 'NONE', #18040, #17256, #20008, .T. ) ;
#5795=CARTESIAN_POINT ( 'NONE',  ( 43.81608638205700146, 0.9984178969752143251, 11.59873562314662010 ) ) ;
#5816=LINE ( 'NONE', #3741, #10181 ) ;
#5823=CARTESIAN_POINT ( 'NONE',  ( 34.06606138205700773, 3.151453266960317023, 6.397347472316774031 ) ) ;
#5843=ORIENTED_EDGE ( 'NONE', *, *, #9409, .T. ) ;
#5873=VERTEX_POINT ( 'NONE', #6766 ) ;
#5879=ORIENTED_EDGE ( 'NONE', *, *, #17907, .T. ) ;
#5902=CARTESIAN_POINT ( 'NONE',  ( 43.69896204258590444, 3.548173818309678484, 6.215045287937394747 ) ) ;
#5912=AXIS2_PLACEMENT_3D ( 'NONE', #9580, #1687, #9454 ) ;
#5926=CARTESIAN_POINT ( 'NONE',  ( 32.81606138205700773, 2.740850673309605412, 6.112030963703427133 ) ) ;
#5941=EDGE_CURVE ( 'NONE', #22555, #9175, #22468, .T. ) ;
#5979=DIRECTION ( 'NONE',  ( -1.849283715844614702E-16, 0.8212051873014210024, 0.5706330172266920187 ) ) ;
#5983=DIRECTION ( 'NONE',  ( 0.000000000000000000, -0.8212051873014208914, -0.5706330172266919076 ) ) ;
#6010=CARTESIAN_POINT ( 'NONE',  ( 32.82453666081570276, -33.17626767724735259, 59.69730752409159180 ) ) ;
#6024=CARTESIAN_POINT ( 'NONE',  ( 43.31606138205700063, -35.82531359714782582, 71.25150419970752580 ) ) ;
#6045=DIRECTION ( 'NONE',  ( -1.000000000000000000, 0.000000000000000000, 0.000000000000000000 ) ) ;
#6046=CIRCLE ( 'NONE', #20442, 2.500000000000002220 ) ;
#6052=DIRECTION ( 'NONE',  ( 1.000000000000000000, -2.616121358439845201E-18, 3.764893311995947332E-18 ) ) ;
#6057=FACE_OUTER_BOUND ( 'NONE', #21026, .T. ) ;
#6063=ORIENTED_EDGE ( 'NONE', *, *, #23181, .T. ) ;
#6087=CARTESIAN_POINT ( 'NONE',  ( 32.81606138205700773, -33.70281195181703993, 69.07320514641659770 ) ) ;
#6098=ORIENTED_EDGE ( 'NONE', *, *, #4521, .F. ) ;
#6108=ORIENTED_EDGE ( 'NONE', *, *, #24822, .T. ) ;
#6109=CARTESIAN_POINT ( 'NONE',  ( 33.48762233684214351, 2.904852044443344106, 6.096108814113431862 ) ) ;
#6152=AXIS2_PLACEMENT_3D ( 'NONE', #11733, #19432, #13523 ) ;
#6154=FACE_BOUND ( 'NONE', #12545, .T. ) ;
#6161=ORIENTED_EDGE ( 'NONE', *, *, #4833, .F. ) ;
#6166=AXIS2_PLACEMENT_3D ( 'NONE', #8834, #3396, #11275 ) ;
#6171=VECTOR ( 'NONE', #19324, 1000.000000000000114 ) ;
#6185=ORIENTED_EDGE ( 'NONE', *, *, #22647, .F. ) ;
#6198=ORIENTED_EDGE ( 'NONE', *, *, #19626, .F. ) ;
#6231=FACE_OUTER_BOUND ( 'NONE', #13717, .T. ) ;
#6246=DIRECTION ( 'NONE',  ( 0.3420484745865489673, -0.7716719862102489058, -0.5362137509718902795 ) ) ;
#6258=DIRECTION ( 'NONE',  ( -1.849283715844614456E-16, 0.8212051873014208914, 0.5706330172266919076 ) ) ;
#6280=DIRECTION ( 'NONE',  ( 1.000000000000000000, 0.000000000000000000, 0.000000000000000000 ) ) ;
#6298=CARTESIAN_POINT ( 'NONE',  ( 43.31606138205700063, 2.476587234117772596, 12.62587505415466538 ) ) ;
#6311=CARTESIAN_POINT ( 'NONE',  ( 32.81606138205700773, -35.41471100349711065, 71.53682070832086026 ) ) ;
#6313=ORIENTED_EDGE ( 'NONE', *, *, #11618, .F. ) ;
#6325=ORIENTED_EDGE ( 'NONE', *, *, #12714, .F. ) ;
#6357=CIRCLE ( 'NONE', #20752, 0.7499999999999983347 ) ;
#6370=CARTESIAN_POINT ( 'NONE',  ( 33.72038411900482657, 3.276404855341859879, 6.354292672467103387 ) ) ;
#6380=LINE ( 'NONE', #14356, #23430 ) ;
#6381=ORIENTED_EDGE ( 'NONE', *, *, #1316, .F. ) ;
#6392=LINE ( 'NONE', #4458, #21908 ) ;
#6393=ORIENTED_EDGE ( 'NONE', *, *, #3919, .T. ) ;
#6394=CARTESIAN_POINT ( 'NONE',  ( 32.81606138205700773, 2.476587234117772596, 12.62587505415466538 ) ) ;
#6413=EDGE_CURVE ( 'NONE', #23317, #13033, #20898, .T. ) ;
#6418=EDGE_LOOP ( 'NONE', ( #15073, #3149, #24540, #6768 ) ) ;
#6426=ADVANCED_FACE ( 'NONE', ( #16645, #17037, #14836 ), #5187, .F. ) ;
#6429=CARTESIAN_POINT ( 'NONE',  ( 32.99554091088185714, 3.410282305729706032, 6.167518378462459872 ) ) ;
#6430=DIRECTION ( 'NONE',  ( 1.000000000000000000, -1.582848796673007376E-16, -1.099878323500689822E-16 ) ) ;
#6432=DIRECTION ( 'NONE',  ( 0.000000000000000000, -0.5706330172266920187, 0.8212051873014210024 ) ) ;
#6438=FACE_OUTER_BOUND ( 'NONE', #19775, .T. ) ;
#6449=DIRECTION ( 'NONE',  ( 0.000000000000000000, 0.9038432971286278761, 0.4278636397681519488 ) ) ;
#6452=DIRECTION ( 'NONE',  ( 0.000000000000000000, 0.8212051873014223347, 0.5706330172266899092 ) ) ;
#6453=DIRECTION ( 'NONE',  ( -1.000000000000000000, 0.000000000000000000, 0.000000000000000000 ) ) ;
#6498=VERTEX_POINT ( 'NONE', #10733 ) ;
#6509=EDGE_LOOP ( 'NONE', ( #11407, #17313 ) ) ;
#6548=DIRECTION ( 'NONE',  ( 0.000000000000000000, 0.8212051873014252212, 0.5706330172266858014 ) ) ;
#6550=CARTESIAN_POINT ( 'NONE',  ( 43.24580177837434292, 3.721690752961227755, 6.335617458560805382 ) ) ;
#6552=CARTESIAN_POINT ( 'NONE',  ( 43.24580177837434292, 3.721690752961224202, 6.335617458560805382 ) ) ;
#6555=EDGE_LOOP ( 'NONE', ( #16737, #24347, #19049, #22315 ) ) ;
#6575=CARTESIAN_POINT ( 'NONE',  ( 43.81606138205700063, -27.17722769842920272, 59.42551550655435477 ) ) ;
#6578=ADVANCED_FACE ( 'NONE', ( #9565, #21532 ), #9816, .T. ) ;
#6583=CARTESIAN_POINT ( 'NONE',  ( 43.81606138205700063, -40.62725863591898445, 68.52362519861142687 ) ) ;
#6584=CIRCLE ( 'NONE', #21391, 0.5000000000000008882 ) ;
#6606=DIRECTION ( 'NONE',  ( 0.000000000000000000, 0.1771812806364704007, 0.9841782327363373106 ) ) ;
#6610=ORIENTED_EDGE ( 'NONE', *, *, #16304, .T. ) ;
#6624=VERTEX_POINT ( 'NONE', #13799 ) ;
#6625=ORIENTED_EDGE ( 'NONE', *, *, #20805, .F. ) ;
#6642=AXIS2_PLACEMENT_3D ( 'NONE', #23896, #2259, #16290 ) ;
#6643=VERTEX_POINT ( 'NONE', #15345 ) ;
#6680=VECTOR ( 'NONE', #22768, 1000.000000000000000 ) ;
#6688=AXIS2_PLACEMENT_3D ( 'NONE', #1090, #22617, #22741 ) ;
#6727=ADVANCED_FACE ( 'NONE', ( #12521 ), #8128, .T. ) ;
#6740=ADVANCED_FACE ( 'NONE', ( #24078 ), #10570, .F. ) ;
#6753=DIRECTION ( 'NONE',  ( -0.9797958971132711969, -0.1642410374602840950, -0.1141266034453383288 ) ) ;
#6754=ORIENTED_EDGE ( 'NONE', *, *, #16616, .F. ) ;
#6765=VERTEX_POINT ( 'NONE', #12387 ) ;
#6766=CARTESIAN_POINT ( 'NONE',  ( 42.56606138205700063, -33.36905983554797217, 58.95447945960771818 ) ) ;
#6768=ORIENTED_EDGE ( 'NONE', *, *, #18408, .T. ) ;
#6791=VERTEX_POINT ( 'NONE', #8512 ) ;
#6803=DIRECTION ( 'NONE',  ( -1.000000000000000000, -1.148292460158763848E-16, -7.979170143241527150E-17 ) ) ;
#6811=CARTESIAN_POINT ( 'NONE',  ( 33.33121445922205339, -32.87633672316712108, 59.29685926994373091 ) ) ;
#6813=CARTESIAN_POINT ( 'NONE',  ( 32.81606138205700773, -27.17722769842920272, 59.42551550655435477 ) ) ;
#6814=ORIENTED_EDGE ( 'NONE', *, *, #22457, .T. ) ;
#6816=DIRECTION ( 'NONE',  ( 1.000000000000000000, -1.717186273645140974E-30, 2.471224469859308882E-30 ) ) ;
#6828=DIRECTION ( 'NONE',  ( 0.000000000000000000, -0.5706330172266952383, 0.8212051873014186709 ) ) ;
#6851=LINE ( 'NONE', #22442, #2168 ) ;
#6893=DIRECTION ( 'NONE',  ( 0.9063205284231096170, -0.3470338693031059241, -0.2411443412468348979 ) ) ;
#6903=EDGE_CURVE ( 'NONE', #1510, #22006, #10515, .T. ) ;
#6921=ORIENTED_EDGE ( 'NONE', *, *, #15258, .T. ) ;
#6930=DIRECTION ( 'NONE',  ( 9.887484856639309956E-17, -0.9841782327363374216, 0.1771812806364704285 ) ) ;
#6936=CARTESIAN_POINT ( 'NONE',  ( 33.31606138205700773, -33.36512800456291217, 60.17493404035838012 ) ) ;
#6957=ORIENTED_EDGE ( 'NONE', *, *, #23871, .F. ) ;
#6981=EDGE_CURVE ( 'NONE', #12466, #25158, #12768, .T. ) ;
#6983=EDGE_CURVE ( 'NONE', #14092, #20720, #18935, .T. ) ;
#6986=DIRECTION ( 'NONE',  ( -1.000000000000000000, -1.518641380243644581E-16, -1.055262346480601087E-16 ) ) ;
#7003=DIRECTION ( 'NONE',  ( 4.584595141645219056E-18, 0.5706330172266919076, -0.8212051873014208914 ) ) ;
#7008=EDGE_LOOP ( 'NONE', ( #4799, #16892, #22140, #6198 ) ) ;
#7015=ORIENTED_EDGE ( 'NONE', *, *, #25189, .F. ) ;
#7017=CARTESIAN_POINT ( 'NONE',  ( 43.82106138205700319, 3.913219763917289651, 6.295309157738977035 ) ) ;
#7021=CYLINDRICAL_SURFACE ( 'NONE', #2225, 0.5000000000000004441 ) ;
#7023=EDGE_LOOP ( 'NONE', ( #20987, #2869, #13300, #19655 ) ) ;
#7041=CARTESIAN_POINT ( 'NONE',  ( 43.81606138205700063, -33.60910547091194900, 60.61426200347987248 ) ) ;
#7047=ORIENTED_EDGE ( 'NONE', *, *, #19037, .T. ) ;
#7057=ORIENTED_EDGE ( 'NONE', *, *, #15856, .F. ) ;
#7061=EDGE_CURVE ( 'NONE', #10887, #5392, #13775, .T. ) ;
#7063=CARTESIAN_POINT ( 'NONE',  ( 43.39709375099387501, 3.108381023609330107, 6.137326095127796144 ) ) ;
#7064=LINE ( 'NONE', #22650, #15950 ) ;
#7096=CARTESIAN_POINT ( 'NONE',  ( 34.06606138205700773, -33.36905983554797217, 58.95447945960771818 ) ) ;
#7133=CARTESIAN_POINT ( 'NONE',  ( 43.31606138205700063, 4.103895195095678794, 6.341006091748962348 ) ) ;
#7141=CARTESIAN_POINT ( 'NONE',  ( 33.56861364504067069, 3.414468223740623642, 6.349533009087196866 ) ) ;
#7148=EDGE_CURVE ( 'NONE', #18371, #7627, #861, .T. ) ;
#7149=AXIS2_PLACEMENT_3D ( 'NONE', #18180, #8513, #134 ) ;
#7154=DIRECTION ( 'NONE',  ( 0.000000000000000000, -0.8212051873014203363, -0.5706330172266926848 ) ) ;
#7162=ORIENTED_EDGE ( 'NONE', *, *, #1040, .T. ) ;
#7175=ORIENTED_EDGE ( 'NONE', *, *, #699, .T. ) ;
#7177=CARTESIAN_POINT ( 'NONE',  ( 32.81606138205700773, 6.294683054830111146, 7.131205101789720224 ) ) ;
#7178=CARTESIAN_POINT ( 'NONE',  ( 43.38751061443460344, 3.099069811988895751, 6.135932541694130826 ) ) ;
#7189=VECTOR ( 'NONE', #20009, 1000.000000000000000 ) ;
#7192=ORIENTED_EDGE ( 'NONE', *, *, #1040, .F. ) ;
#7198=DIRECTION ( 'NONE',  ( -1.292986538149619279E-16, 0.9897030922575080769, 0.1431355622335914179 ) ) ;
#7213=ORIENTED_EDGE ( 'NONE', *, *, #17127, .F. ) ;
#7258=LINE ( 'NONE', #7133, #18478 ) ;
#7275=EDGE_CURVE ( 'NONE', #19784, #18363, #10161, .T. ) ;
#7276=ADVANCED_FACE ( 'NONE', ( #12362 ), #2536, .F. ) ;
#7289=CARTESIAN_POINT ( 'NONE',  ( 43.31097620093147071, -33.12114940777929917, 59.73560686274496589 ) ) ;
#7293=CARTESIAN_POINT ( 'NONE',  ( 43.30090830489194786, -32.87633672316712108, 59.29685926994373091 ) ) ;
#7298=AXIS2_PLACEMENT_3D ( 'NONE', #23201, #15602, #3750 ) ;
#7303=VECTOR ( 'NONE', #1882, 1000.000000000000114 ) ;
#7310=CARTESIAN_POINT ( 'NONE',  ( 42.56606138205700063, 2.740850673309605412, 6.112030963703427133 ) ) ;
#7312=ORIENTED_EDGE ( 'NONE', *, *, #18005, .F. ) ;
#7313=ORIENTED_EDGE ( 'NONE', *, *, #21868, .F. ) ;
#7314=CARTESIAN_POINT ( 'NONE',  ( 43.39709375099424449, 3.108381023609659621, 6.137326095127897396 ) ) ;
#7317=FACE_OUTER_BOUND ( 'NONE', #20049, .T. ) ;
#7319=AXIS2_PLACEMENT_3D ( 'NONE', #12752, #18919, #12270 ) ;
#7328=VERTEX_POINT ( 'NONE', #6298 ) ;
#7346=EDGE_CURVE ( 'NONE', #4607, #5873, #10416, .T. ) ;
#7364=EDGE_CURVE ( 'NONE', #13605, #2134, #853, .T. ) ;
#7377=CARTESIAN_POINT ( 'NONE',  ( 32.81606138205700773, 0.9984178969752143251, 11.59873562314662010 ) ) ;
#7383=DIRECTION ( 'NONE',  ( 0.000000000000000000, 0.5706330172266952383, -0.8212051873014186709 ) ) ;
#7388=PLANE ( 'NONE',  #5912 ) ;
#7407=CARTESIAN_POINT ( 'NONE',  ( 43.81606138205700063, 6.289375473607850431, 7.138843309009015314 ) ) ;
#7415=ORIENTED_EDGE ( 'NONE', *, *, #4994, .F. ) ;
#7421=ORIENTED_EDGE ( 'NONE', *, *, #23881, .T. ) ;
#7423=AXIS2_PLACEMENT_3D ( 'NONE', #24972, #14354, #20529 ) ;
#7424=CARTESIAN_POINT ( 'NONE',  ( 43.31606138205700063, -33.36512788127016904, 60.17493381834628252 ) ) ;
#7430=CARTESIAN_POINT ( 'NONE',  ( 43.31606138205700063, -0.03546393544221274063, 20.62209909563275900 ) ) ;
#7455=ORIENTED_EDGE ( 'NONE', *, *, #15389, .F. ) ;
#7463=CARTESIAN_POINT ( 'NONE',  ( 33.48998873999627079, 2.908502444426765532, 6.098666494912968972 ) ) ;
#7478=CYLINDRICAL_SURFACE ( 'NONE', #13183, 0.4999999999999982792 ) ;
#7490=ORIENTED_EDGE ( 'NONE', *, *, #18033, .T. ) ;
#7497=DIRECTION ( 'NONE',  ( 0.000000000000000000, -0.5706330172266952383, 0.8212051873014186709 ) ) ;
#7506=CARTESIAN_POINT ( 'NONE',  ( 33.42807400205546742, 3.632122393466618249, 6.321668986087207287 ) ) ;
#7521=VECTOR ( 'NONE', #18282, 1000.000000000000114 ) ;
#7548=ORIENTED_EDGE ( 'NONE', *, *, #22457, .F. ) ;
#7556=ADVANCED_FACE ( 'NONE', ( #21471 ), #3736, .T. ) ;
#7569=CARTESIAN_POINT ( 'NONE',  ( 33.31606138205700773, -33.60910547091194900, 60.61426200347987248 ) ) ;
#7573=B_SPLINE_CURVE_WITH_KNOTS ( 'NONE', 3,
 ( #13810, #14201, #10327, #4405, #4018, #20116, #3894, #2207, #21548, #18189 ),
 .UNSPECIFIED., .F., .F.,
 ( 4, 3, 3, 4 ),
 ( 2.611104600503255186E-18, 0.0001276540846395581876, 0.0002420623083067835056, 0.0003579128776106695184 ),
 .UNSPECIFIED. ) ;
#7576=VECTOR ( 'NONE', #18758, 1000.000000000000000 ) ;
#7602=EDGE_CURVE ( 'NONE', #10132, #19839, #11437, .T. ) ;
#7613=ORIENTED_EDGE ( 'NONE', *, *, #11384, .T. ) ;
#7615=B_SPLINE_CURVE_WITH_KNOTS ( 'NONE', 3,
 ( #17749, #81, #9766, #3827 ),
 .UNSPECIFIED., .F., .F.,
 ( 4, 4 ),
 ( 0.000000000000000000, 1.000000000000000000 ),
 .UNSPECIFIED. ) ;
#7617=ORIENTED_EDGE ( 'NONE', *, *, #24822, .F. ) ;
#7627=VERTEX_POINT ( 'NONE', #24925 ) ;
#7631=LINE ( 'NONE', #9569, #8234 ) ;
#7634=CARTESIAN_POINT ( 'NONE',  ( 34.06606138205700773, 2.740850673309605412, 6.112030963703427133 ) ) ;
#7641=CARTESIAN_POINT ( 'NONE',  ( 33.23058527440274190, 3.113468987225101348, 6.136968036621309963 ) ) ;
#7643=LINE ( 'NONE', #23335, #24205 ) ;
#7666=ORIENTED_EDGE ( 'NONE', *, *, #7061, .F. ) ;
#7672=ORIENTED_EDGE ( 'NONE', *, *, #7843, .T. ) ;
#7688=CARTESIAN_POINT ( 'NONE',  ( 32.81606138205700773, -33.60910547091194900, 60.61426200347987248 ) ) ;
#7692=EDGE_CURVE ( 'NONE', #5392, #10132, #8078, .T. ) ;
#7704=LINE ( 'NONE', #5769, #25422 ) ;
#7719=ORIENTED_EDGE ( 'NONE', *, *, #17127, .T. ) ;
#7720=CARTESIAN_POINT ( 'NONE',  ( 33.35563295957085472, 2.997420204183892434, 6.110946949555683183 ) ) ;
#7721=LINE ( 'NONE', #1898, #8815 ) ;
#7726=AXIS2_PLACEMENT_3D ( 'NONE', #8866, #1240, #9122 ) ;
#7742=B_SPLINE_CURVE_WITH_KNOTS ( 'NONE', 3,
 ( #644, #18192, #16626, #20372 ),
 .UNSPECIFIED., .F., .F.,
 ( 4, 4 ),
 ( 0.000000000000000000, 1.000000000000000000 ),
 .UNSPECIFIED. ) ;
#7765=CARTESIAN_POINT ( 'NONE',  ( 32.84837986530673248, 3.753595868030215499, 6.230380467512803833 ) ) ;
#7766=AXIS2_PLACEMENT_3D ( 'NONE', #19307, #15569, #100 ) ;
#7793=AXIS2_PLACEMENT_3D ( 'NONE', #21764, #21893, #12505 ) ;
#7801=ORIENTED_EDGE ( 'NONE', *, *, #17489, .F. ) ;
#7808=CARTESIAN_POINT ( 'NONE',  ( 32.81606138205700773, -27.60498114914039647, 57.04949906928989378 ) ) ;
#7815=ORIENTED_EDGE ( 'NONE', *, *, #16885, .T. ) ;
#7823=CARTESIAN_POINT ( 'NONE',  ( 42.65336712727322777, 3.163553052512885877, 6.379934517999310550 ) ) ;
#7830=CARTESIAN_POINT ( 'NONE',  ( 43.31606138205700063, 2.476587234117772596, 12.62587505415466538 ) ) ;
#7831=FACE_OUTER_BOUND ( 'NONE', #12456, .T. ) ;
#7843=EDGE_CURVE ( 'NONE', #5208, #4227, #9194, .T. ) ;
#7878=VERTEX_POINT ( 'NONE', #5566 ) ;
#7889=PLANE ( 'NONE',  #7298 ) ;
#7901=PLANE ( 'NONE',  #11409 ) ;
#7902=CIRCLE ( 'NONE', #22270, 0.4999999999999982792 ) ;
#7915=SURFACE_SIDE_STYLE ('',( #8844 ) ) ;
#7918=PLANE ( 'NONE',  #20475 ) ;
#7919=AXIS2_PLACEMENT_3D ( 'NONE', #9006, #16853, #24435 ) ;
#7920=ORIENTED_EDGE ( 'NONE', *, *, #13378, .F. ) ;
#7924=CARTESIAN_POINT ( 'NONE',  ( 33.63983381732882805, 3.338985100189890254, 6.348312178689752727 ) ) ;
#7934=CARTESIAN_POINT ( 'NONE',  ( 32.81606138205700773, -27.66931681479738003, 59.51410614687260647 ) ) ;
#7942=ORIENTED_EDGE ( 'NONE', *, *, #5648, .F. ) ;
#7948=EDGE_LOOP ( 'NONE', ( #17311, #19488, #6108, #21449 ) ) ;
#7951=CARTESIAN_POINT ( 'NONE',  ( 32.81606138205700773, -33.39268706791821728, 60.15578316240965506 ) ) ;
#7972=CIRCLE ( 'NONE', #1371, 0.5000000000000022204 ) ;
#7975=ORIENTED_EDGE ( 'NONE', *, *, #5626, .T. ) ;
#7982=AXIS2_PLACEMENT_3D ( 'NONE', #6583, #14686, #10960 ) ;
#7983=ORIENTED_EDGE ( 'NONE', *, *, #6903, .F. ) ;
#7990=AXIS2_PLACEMENT_3D ( 'NONE', #5196, #14981, #17778 ) ;
#7993=CARTESIAN_POINT ( 'NONE',  ( 34.06606138205700773, -39.60075215179220720, 69.23691647014479145 ) ) ;
#7995=FACE_OUTER_BOUND ( 'NONE', #13172, .T. ) ;
#8014=CARTESIAN_POINT ( 'NONE',  ( 43.81606138205700063, -34.55876147765707174, 70.30501292736873609 ) ) ;
#8017=DIRECTION ( 'NONE',  ( 0.000000000000000000, 0.5706330172266919076, -0.8212051873014208914 ) ) ;
#8021=EDGE_CURVE ( 'NONE', #23179, #18040, #1677, .T. ) ;
#8023=EDGE_CURVE ( 'NONE', #6791, #12100, #25375, .T. ) ;
#8029=EDGE_CURVE ( 'NONE', #12177, #20637, #7631, .T. ) ;
#8033=EDGE_LOOP ( 'NONE', ( #15489, #24827, #2025, #12207 ) ) ;
#8035=ORIENTED_EDGE ( 'NONE', *, *, #889, .F. ) ;
#8040=EDGE_CURVE ( 'NONE', #20004, #1510, #3884, .T. ) ;
#8062=CARTESIAN_POINT ( 'NONE',  ( 33.31606138205700773, -27.25871422114667553, 59.79942265548595515 ) ) ;
#8078=LINE ( 'NONE', #12076, #22705 ) ;
#8079=CARTESIAN_POINT ( 'NONE',  ( 38.31606138205700063, -29.78523130861184143, 52.92072663988442116 ) ) ;
#8102=CARTESIAN_POINT ( 'NONE',  ( 42.56606138205700063, -32.75315594507191008, 59.38245422252773409 ) ) ;
#8105=CARTESIAN_POINT ( 'NONE',  ( 32.81606138205700773, 4.124002793203064066, 6.312068993173404863 ) ) ;
#8108=CARTESIAN_POINT ( 'NONE',  ( 43.30251437062377562, 3.928705369154989135, 6.336397002151890057 ) ) ;
#8111=DIRECTION ( 'NONE',  ( -1.000000000000000000, 0.000000000000000000, 0.000000000000000000 ) ) ;
#8119=VERTEX_POINT ( 'NONE', #2818 ) ;
#8125=AXIS2_PLACEMENT_3D ( 'NONE', #4068, #11425, #2118 ) ;
#8126=DIRECTION ( 'NONE',  ( 0.000000000000000000, 0.5706330172266920187, -0.8212051873014210024 ) ) ;
#8127=EDGE_LOOP ( 'NONE', ( #8205, #21422, #7313, #12080 ) ) ;
#8128=CYLINDRICAL_SURFACE ( 'NONE', #2271, 0.4999999999999982792 ) ;
#8154=DIRECTION ( 'NONE',  ( 0.000000000000000000, 0.5706330172266919076, -0.8212051873014208914 ) ) ;
#8159=EDGE_CURVE ( 'NONE', #13577, #25244, #20362, .T. ) ;
#8169=EDGE_CURVE ( 'NONE', #23532, #20004, #8254, .T. ) ;
#8183=EDGE_LOOP ( 'NONE', ( #18540, #20030, #23817, #7613, #6063, #23031, #7421, #3796, #12314, #14967, #16575, #22904, #435, #1746, #14732, #15175, #19822, #24588, #9971 ) ) ;
#8186=ORIENTED_EDGE ( 'NONE', *, *, #554, .F. ) ;
#8205=ORIENTED_EDGE ( 'NONE', *, *, #19252, .T. ) ;
#8217=VECTOR ( 'NONE', #855, 1000.000000000000000 ) ;
#8224=CIRCLE ( 'NONE', #17261, 0.4999999999999982792 ) ;
#8234=VECTOR ( 'NONE', #19466, 1000.000000000000000 ) ;
#8235=ADVANCED_FACE ( 'NONE', ( #19983 ), #18055, .F. ) ;
#8236=CARTESIAN_POINT ( 'NONE',  ( 42.82259893474252266, 3.224890024296139135, 6.370941811568299862 ) ) ;
#8237=( NAMED_UNIT ( * ) SI_UNIT ( $, .STERADIAN. ) SOLID_ANGLE_UNIT ( ) );
#8239=CARTESIAN_POINT ( 'NONE',  ( 43.81606138205700063, 3.151453266960317023, 6.397347472316774031 ) ) ;
#8241=PLANE ( 'NONE',  #7793 ) ;
#8254=CIRCLE ( 'NONE', #25081, 0.7499999999999983347 ) ;
#8259=CARTESIAN_POINT ( 'NONE',  ( 34.06606138205700773, -39.60075215179220720, 69.23691647014479145 ) ) ;
#8262=DIRECTION ( 'NONE',  ( -1.000000000000000000, 0.000000000000000000, 0.000000000000000000 ) ) ;
#8289=ORIENTED_EDGE ( 'NONE', *, *, #2231, .F. ) ;
#8333=AXIS2_PLACEMENT_3D ( 'NONE', #7177, #24916, #12849 ) ;
#8342=EDGE_CURVE ( 'NONE', #24513, #6624, #16398, .T. ) ;
#8356=AXIS2_PLACEMENT_3D ( 'NONE', #16981, #13121, #5137 ) ;
#8360=CARTESIAN_POINT ( 'NONE',  ( 43.81606138205700063, -25.26124097814961544, 70.06813202641110649 ) ) ;
#8367=AXIS2_PLACEMENT_3D ( 'NONE', #15123, #4824, #9346 ) ;
#8369=FACE_OUTER_BOUND ( 'NONE', #2459, .T. ) ;
#8380=AXIS2_PLACEMENT_3D ( 'NONE', #2731, #14984, #14598 ) ;
#8388=CARTESIAN_POINT ( 'NONE',  ( 38.31606138205700063, -29.78523130861184143, 52.92072663988442116 ) ) ;
#8422=STYLED_ITEM ( 'NONE', ( #11915 ), #16907 ) ;
#8429=DIRECTION ( 'NONE',  ( 1.000000000000000000, -0.000000000000000000, 0.000000000000000000 ) ) ;
#8437=DIRECTION ( 'NONE',  ( -1.000000000000000000, -1.208430656372714685E-15, -2.875977885193763990E-16 ) ) ;
#8460=VERTEX_POINT ( 'NONE', #2039 ) ;
#8463=DIRECTION ( 'NONE',  ( 1.000000000000000000, -0.000000000000000000, 0.000000000000000000 ) ) ;
#8477=ADVANCED_FACE ( 'NONE', ( #25344 ), #17775, .F. ) ;
#8494=ADVANCED_FACE ( 'NONE', ( #23928 ), #15682, .T. ) ;
#8495=CARTESIAN_POINT ( 'NONE',  ( 43.28398221755340103, 3.843662888489567830, 6.335227539316586665 ) ) ;
#8497=FACE_OUTER_BOUND ( 'NONE', #3081, .T. ) ;
#8512=CARTESIAN_POINT ( 'NONE',  ( 43.81606138205700063, -27.60498114914042134, 57.04949906928994352 ) ) ;
#8513=DIRECTION ( 'NONE',  ( 1.000000000000000000, -0.000000000000000000, 0.000000000000000000 ) ) ;
#8521=CARTESIAN_POINT ( 'NONE',  ( 32.81606138205700773, 2.887189827768484207, 12.91119156276801228 ) ) ;
#8531=CIRCLE ( 'NONE', #16741, 0.4999999999999943379 ) ;
#8535=AXIS2_PLACEMENT_3D ( 'NONE', #15617, #15870, #18073 ) ;
#8560=EDGE_CURVE ( 'NONE', #18636, #2353, #24057, .T. ) ;
#8598=VECTOR ( 'NONE', #230, 1000.000000000000000 ) ;
#8615=CARTESIAN_POINT ( 'NONE',  ( 43.38751330861478550, 3.099072278388469659, 6.135933108610706732 ) ) ;
#8617=CARTESIAN_POINT ( 'NONE',  ( 34.06606138205700773, 2.740850673309605412, 6.112030963703427133 ) ) ;
#8621=EDGE_CURVE ( 'NONE', #4551, #19784, #16855, .T. ) ;
#8648=ORIENTED_EDGE ( 'NONE', *, *, #21347, .F. ) ;
#8651=CARTESIAN_POINT ( 'NONE',  ( 43.81608638205700146, 2.761903742731119049, 12.21527246050395377 ) ) ;
#8658=DIRECTION ( 'NONE',  ( 1.000000000000000000, -0.000000000000000000, 0.000000000000000000 ) ) ;
#8665=ORIENTED_EDGE ( 'NONE', *, *, #21878, .F. ) ;
#8672=ORIENTED_EDGE ( 'NONE', *, *, #21067, .F. ) ;
#8699=ORIENTED_EDGE ( 'NONE', *, *, #9409, .F. ) ;
#8708=VERTEX_POINT ( 'NONE', #20457 ) ;
#8714=EDGE_CURVE ( 'NONE', #13705, #24513, #12993, .T. ) ;
#8749=CARTESIAN_POINT ( 'NONE',  ( 43.62721312654221606, 3.386191220328446772, 6.178494284004524495 ) ) ;
#8751=ADVANCED_FACE ( 'NONE', ( #14906 ), #24812, .F. ) ;
#8761=UNCERTAINTY_MEASURE_WITH_UNIT (LENGTH_MEASURE( 1.000000000000000082E-05 ), #21579, 'distance_accuracy_value', 'NONE');
#8777=CARTESIAN_POINT ( 'NONE',  ( 32.81606138205700773, 6.366250835946940967, 6.636353555660927661 ) ) ;
#8779=CARTESIAN_POINT ( 'NONE',  ( 32.81606138205700773, -27.25871422114667553, 59.79942265548595515 ) ) ;
#8804=ORIENTED_EDGE ( 'NONE', *, *, #22249, .T. ) ;
#8815=VECTOR ( 'NONE', #9785, 1000.000000000000114 ) ;
#8822=CARTESIAN_POINT ( 'NONE',  ( 33.56861364504118228, 3.414468223740023234, 6.349533009087269697 ) ) ;
#8834=CARTESIAN_POINT ( 'NONE',  ( 42.56606138205700063, -32.75315594507191008, 59.38245422252773409 ) ) ;
#8844=SURFACE_STYLE_FILL_AREA ( #19247 ) ;
#8858=DIRECTION ( 'NONE',  ( 1.000000000000000000, 0.000000000000000000, 0.000000000000000000 ) ) ;
#8866=CARTESIAN_POINT ( 'NONE',  ( 43.81606138205700063, 2.761903742731119049, 12.21527246050395377 ) ) ;
#8889=ORIENTED_EDGE ( 'NONE', *, *, #18613, .F. ) ;
#8905=DIRECTION ( 'NONE',  ( -1.000000000000000000, -7.979170143241514824E-17, 1.148292460158762122E-16 ) ) ;
#8909=PLANE ( 'NONE',  #7982 ) ;
#8922=ORIENTED_EDGE ( 'NONE', *, *, #23181, .F. ) ;
#8942=ADVANCED_FACE ( 'NONE', ( #13553, #8 ), #7889, .T. ) ;
#8951=CARTESIAN_POINT ( 'NONE',  ( 33.56477571746443544, 3.418883076854447367, 6.349191931652266696 ) ) ;
#8967=CYLINDRICAL_SURFACE ( 'NONE', #5673, 0.4999999999999998890 ) ;
#8979=LINE ( 'NONE', #22620, #7576 ) ;
#8996=DIRECTION ( 'NONE',  ( 0.000000000000000000, -0.5706330172266919076, 0.8212051873014208914 ) ) ;
#9006=CARTESIAN_POINT ( 'NONE',  ( 32.81606138205700773, -34.55876147765707174, 70.30501292736873609 ) ) ;
#9007=CARTESIAN_POINT ( 'NONE',  ( 40.56606138205700773, 5.719301844480432884, 2.701924129460374413 ) ) ;
#9015=ORIENTED_EDGE ( 'NONE', *, *, #8159, .T. ) ;
#9023=DIRECTION ( 'NONE',  ( 0.000000000000000000, -0.8212051873014252212, -0.5706330172266858014 ) ) ;
#9029=ORIENTED_EDGE ( 'NONE', *, *, #16831, .T. ) ;
#9034=ADVANCED_FACE ( 'NONE', ( #2069 ), #13415, .T. ) ;
#9043=CIRCLE ( 'NONE', #14364, 0.5000000000000004441 ) ;
#9046=ORIENTED_EDGE ( 'NONE', *, *, #13974, .T. ) ;
#9053=VECTOR ( 'NONE', #12365, 1000.000000000000114 ) ;
#9064=DIRECTION ( 'NONE',  ( -1.000000000000000000, 0.000000000000000000, 0.000000000000000000 ) ) ;
#9080=FACE_OUTER_BOUND ( 'NONE', #5748, .T. ) ;
#9087=VERTEX_POINT ( 'NONE', #6575 ) ;
#9095=CARTESIAN_POINT ( 'NONE',  ( 43.29192581567074427, 3.843594479409538689, 6.333537542383846031 ) ) ;
#9104=VERTEX_POINT ( 'NONE', #10197 ) ;
#9122=DIRECTION ( 'NONE',  ( 0.000000000000000000, -0.5706330172266930179, 0.8212051873014202252 ) ) ;
#9126=ORIENTED_EDGE ( 'NONE', *, *, #25130, .T. ) ;
#9130=CIRCLE ( 'NONE', #13246, 0.5000000000000004441 ) ;
#9140=CARTESIAN_POINT ( 'NONE',  ( 32.81606138205700773, -30.89740888249930961, 1.247106086993583718 ) ) ;
#9143=LINE ( 'NONE', #1262, #1588 ) ;
#9152=CARTESIAN_POINT ( 'NONE',  ( 42.82259893474252266, 3.224890024296139135, 6.370941811568299862 ) ) ;
#9175=VERTEX_POINT ( 'NONE', #12263 ) ;
#9189=EDGE_LOOP ( 'NONE', ( #2656, #16819, #8665, #2961 ) ) ;
#9194=LINE ( 'NONE', #14709, #4204 ) ;
#9207=FACE_OUTER_BOUND ( 'NONE', #14100, .T. ) ;
#9218=CARTESIAN_POINT ( 'NONE',  ( 33.57054579126888427, 3.412273012123826721, 6.349712035633041651 ) ) ;
#9237=MECHANICAL_DESIGN_GEOMETRIC_PRESENTATION_REPRESENTATION('',(#22379),#10046);
#9242=CARTESIAN_POINT ( 'NONE',  ( 43.31606138205700063, -1.963190818658398173, 19.89143565483009013 ) ) ;
#9248=ORIENTED_EDGE ( 'NONE', *, *, #11453, .T. ) ;
#9250=ORIENTED_EDGE ( 'NONE', *, *, #20098, .T. ) ;
#9257=ORIENTED_EDGE ( 'NONE', *, *, #8342, .F. ) ;
#9263=AXIS2_PLACEMENT_3D ( 'NONE', #2600, #16514, #4308 ) ;
#9267=CARTESIAN_POINT ( 'NONE',  ( 43.06085722964723317, 3.410734704100585546, 6.350806999483399551 ) ) ;
#9272=AXIS2_PLACEMENT_3D ( 'NONE', #24987, #3108, #6986 ) ;
#9274=EDGE_CURVE ( 'NONE', #24765, #4360, #1412, .T. ) ;
#9275=ORIENTED_EDGE ( 'NONE', *, *, #19037, .F. ) ;
#9279=ORIENTED_EDGE ( 'NONE', *, *, #20305, .T. ) ;
#9286=CARTESIAN_POINT ( 'NONE',  ( 0.000000000000000000, 0.000000000000000000, 0.000000000000000000 ) ) ;
#9296=CARTESIAN_POINT ( 'NONE',  ( 33.31606138205700773, -37.98241563432386414, 69.85268917996594951 ) ) ;
#9306=ORIENTED_EDGE ( 'NONE', *, *, #18613, .T. ) ;
#9314=FACE_OUTER_BOUND ( 'NONE', #21895, .T. ) ;
#9317=ORIENTED_EDGE ( 'NONE', *, *, #18614, .T. ) ;
#9318=DIRECTION ( 'NONE',  ( 1.000000000000000000, 1.187136597504755470E-16, 8.249087426255173666E-17 ) ) ;
#9331=CARTESIAN_POINT ( 'NONE',  ( 32.81106138205699807, 3.938725376308748416, 6.271190958417212968 ) ) ;
#9341=CARTESIAN_POINT ( 'NONE',  ( 43.81606138205700063, -25.26124097814961544, 70.06813202641110649 ) ) ;
#9346=DIRECTION ( 'NONE',  ( 0.000000000000000000, -0.8212051873014223347, -0.5706330172266899092 ) ) ;
#9349=DIRECTION ( 'NONE',  ( 0.000000000000000000, -0.4278636397681519488, 0.9038432971286277651 ) ) ;
#9351=VECTOR ( 'NONE', #25298, 1000.000000000000000 ) ;
#9358=CARTESIAN_POINT ( 'NONE',  ( 34.06606138205700773, -33.77966242919868733, 58.66916295099436951 ) ) ;
#9382=ORIENTED_EDGE ( 'NONE', *, *, #9662, .T. ) ;
#9398=ORIENTED_EDGE ( 'NONE', *, *, #699, .F. ) ;
#9402=AXIS2_PLACEMENT_3D ( 'NONE', #15020, #18632, #8858 ) ;
#9409=EDGE_CURVE ( 'NONE', #17862, #19940, #5161, .T. ) ;
#9413=EDGE_CURVE ( 'NONE', #5392, #5873, #1146, .T. ) ;
#9427=EDGE_LOOP ( 'NONE', ( #11920, #7548 ) ) ;
#9454=DIRECTION ( 'NONE',  ( 0.000000000000000000, 0.8212051873014208914, 0.5706330172266919076 ) ) ;
#9466=LINE ( 'NONE', #9341, #4258 ) ;
#9468=VECTOR ( 'NONE', #11393, 1000.000000000000000 ) ;
#9471=VERTEX_POINT ( 'NONE', #23170 ) ;
#9477=DIRECTION ( 'NONE',  ( 0.000000000000000000, -0.5706330172266920187, 0.8212051873014210024 ) ) ;
#9481=CARTESIAN_POINT ( 'NONE',  ( 34.06606138205689405, 3.151453266960317023, 6.397347472316774031 ) ) ;
#9488=AXIS2_PLACEMENT_3D ( 'NONE', #5266, #11066, #5394 ) ;
#9493=B_SPLINE_CURVE_WITH_KNOTS ( 'NONE', 3,
 ( #3786, #19010, #11540, #9481 ),
 .UNSPECIFIED., .F., .F.,
 ( 4, 4 ),
 ( 0.000000000000000000, 1.000000000000000000 ),
 .UNSPECIFIED. ) ;
#9495=CARTESIAN_POINT ( 'NONE',  ( 43.31606138205700063, -35.41471100349711065, 71.53682070832086026 ) ) ;
#9510=CIRCLE ( 'NONE', #21827, 0.5000000000000004441 ) ;
#9517=EDGE_CURVE ( 'NONE', #20815, #5873, #3852, .T. ) ;
#9550=EDGE_LOOP ( 'NONE', ( #156, #23917, #1735, #7617 ) ) ;
#9565=FACE_BOUND ( 'NONE', #18696, .T. ) ;
#9569=CARTESIAN_POINT ( 'NONE',  ( 43.31606138205700063, -27.25871422114667553, 59.79942265548595515 ) ) ;
#9580=CARTESIAN_POINT ( 'NONE',  ( 43.81608638205700146, 2.887189827768484207, 12.91119156276801228 ) ) ;
#9588=B_SPLINE_CURVE_WITH_KNOTS ( 'NONE', 3,
 ( #19962, #23935, #23433, #25485 ),
 .UNSPECIFIED., .F., .F.,
 ( 4, 4 ),
 ( 0.0003110653709002429907, 1.000000000000000000 ),
 .UNSPECIFIED. ) ;
#9619=ADVANCED_FACE ( 'NONE', ( #20340 ), #23683, .T. ) ;
#9625=CIRCLE ( 'NONE', #7149, 1.499999999999996669 ) ;
#9626=LINE ( 'NONE', #7808, #20202 ) ;
#9629=DIRECTION ( 'NONE',  ( 0.000000000000000000, -0.8212051873014208914, -0.5706330172266919076 ) ) ;
#9633=AXIS2_PLACEMENT_3D ( 'NONE', #14718, #10617, #926 ) ;
#9637=ORIENTED_EDGE ( 'NONE', *, *, #17291, .F. ) ;
#9647=FACE_OUTER_BOUND ( 'NONE', #2402, .T. ) ;
#9662=EDGE_CURVE ( 'NONE', #2353, #9754, #2206, .T. ) ;
#9663=AXIS2_PLACEMENT_3D ( 'NONE', #13960, #1585, #19504 ) ;
#9667=CARTESIAN_POINT ( 'NONE',  ( 43.81606138205700063, -33.77966242919868733, 58.66916295099436951 ) ) ;
#9693=CARTESIAN_POINT ( 'NONE',  ( 33.31606138205700773, -35.70002751211045933, 71.94742330197156832 ) ) ;
#9734=ADVANCED_FACE ( 'NONE', ( #21758 ), #12116, .T. ) ;
#9735=( NAMED_UNIT ( * ) PLANE_ANGLE_UNIT ( ) SI_UNIT ( $, .RADIAN. ) );
#9738=EDGE_CURVE ( 'NONE', #24709, #10314, #11989, .T. ) ;
#9754=VERTEX_POINT ( 'NONE', #10799 ) ;
#9766=CARTESIAN_POINT ( 'NONE',  ( 43.80758608018112454, -33.17626737717533558, 59.69730689378931032 ) ) ;
#9767=DIRECTION ( 'NONE',  ( -1.000000000000000000, 0.000000000000000000, 0.000000000000000000 ) ) ;
#9773=VECTOR ( 'NONE', #22430, 1000.000000000000114 ) ;
#9775=CARTESIAN_POINT ( 'NONE',  ( 32.84131651066541480, -32.95845724189726411, 59.23979596822106686 ) ) ;
#9782=ORIENTED_EDGE ( 'NONE', *, *, #12099, .F. ) ;
#9784=EDGE_CURVE ( 'NONE', #17728, #9087, #18653, .T. ) ;
#9785=DIRECTION ( 'NONE',  ( 0.000000000000000000, -0.8212051873014208914, -0.5706330172266919076 ) ) ;
#9816=PLANE ( 'NONE',  #19134 ) ;
#9828=DIRECTION ( 'NONE',  ( 1.445602896647340149E-16, -0.8212051873014210024, -0.5706330172266920187 ) ) ;
#9837=ORIENTED_EDGE ( 'NONE', *, *, #20622, .T. ) ;
#9841=VECTOR ( 'NONE', #18982, 1000.000000000000000 ) ;
#9851=CARTESIAN_POINT ( 'NONE',  ( 43.81608638205700146, -1.677874310045055051, 19.48083306117937852 ) ) ;
#9855=CARTESIAN_POINT ( 'NONE',  ( 33.63257508155546560, 2.837830513113499098, 6.099065269017631685 ) ) ;
#9856=CARTESIAN_POINT ( 'NONE',  ( 32.81606138205700773, -37.98241563432386414, 69.85268917996594951 ) ) ;
#9874=ADVANCED_FACE ( 'NONE', ( #14908 ), #14535, .T. ) ;
#9884=EDGE_CURVE ( 'NONE', #13983, #952, #2585, .T. ) ;
#9887=CARTESIAN_POINT ( 'NONE',  ( 43.81606138205700063, -35.41471100349711065, 71.53682070832086026 ) ) ;
#9892=DIRECTION ( 'NONE',  ( 0.000000000000000000, 0.5706330172266907974, -0.8212051873014217795 ) ) ;
#9930=CARTESIAN_POINT ( 'NONE',  ( 42.56606138205700063, -40.21665604226827639, 68.80894170722476133 ) ) ;
#9940=DIRECTION ( 'NONE',  ( 0.000000000000000000, 0.8212051873014208914, 0.5706330172266919076 ) ) ;
#9941=ORIENTED_EDGE ( 'NONE', *, *, #5400, .T. ) ;
#9945=VECTOR ( 'NONE', #19921, 1000.000000000000114 ) ;
#9949=CARTESIAN_POINT ( 'NONE',  ( 33.77108364926073847, 2.783409424099800855, 6.088044787086559495 ) ) ;
#9954=ADVANCED_FACE ( 'NONE', ( #21476 ), #5390, .T. ) ;
#9971=ORIENTED_EDGE ( 'NONE', *, *, #20805, .T. ) ;
#9977=CARTESIAN_POINT ( 'NONE',  ( 34.06606138205700773, -40.21665604226827639, 68.80894170722476133 ) ) ;
#9988=CARTESIAN_POINT ( 'NONE',  ( 43.31606138205700063, -33.60910547091194900, 60.61426200347987248 ) ) ;
#10013=LINE ( 'NONE', #10610, #18629 ) ;
#10026=LINE ( 'NONE', #16061, #10702 ) ;
#10046=( GEOMETRIC_REPRESENTATION_CONTEXT ( 3 ) GLOBAL_UNCERTAINTY_ASSIGNED_CONTEXT ( ( #8761 ) ) GLOBAL_UNIT_ASSIGNED_CONTEXT ( ( #21579, #9735, #11674 ) ) REPRESENTATION_CONTEXT ( 'NONE', 'WORKASPACE' ) );
#10054=CYLINDRICAL_SURFACE ( 'NONE', #3249, 2.500000000000002220 ) ;
#10062=ORIENTED_EDGE ( 'NONE', *, *, #4964, .F. ) ;
#10070=PLANE ( 'NONE',  #4845 ) ;
#10077=CYLINDRICAL_SURFACE ( 'NONE', #15287, 0.4999999999999994449 ) ;
#10109=VECTOR ( 'NONE', #18677, 1000.000000000000000 ) ;
#10130=CARTESIAN_POINT ( 'NONE',  ( 32.81606138205700773, -33.70281195181703993, 69.07320514641659770 ) ) ;
#10132=VERTEX_POINT ( 'NONE', #22233 ) ;
#10143=DIRECTION ( 'NONE',  ( 0.000000000000000000, -0.4278636397681519488, 0.9038432971286277651 ) ) ;
#10148=PRODUCT ( 'Follower', 'Follower', '', ( #21283 ) ) ;
#10151=ORIENTED_EDGE ( 'NONE', *, *, #13378, .T. ) ;
#10154=ORIENTED_EDGE ( 'NONE', *, *, #1042, .T. ) ;
#10155=DIRECTION ( 'NONE',  ( -1.000000000000000000, -1.185941393278724777E-16, -8.240782279085522416E-17 ) ) ;
#10161=LINE ( 'NONE', #14028, #7521 ) ;
#10165=CARTESIAN_POINT ( 'NONE',  ( 43.30787617916693932, 3.971823716557246975, 6.337422814852420316 ) ) ;
#10168=CARTESIAN_POINT ( 'NONE',  ( 32.81606138205700773, -2.373793412309109563, 19.60611914621674146 ) ) ;
#10169=EDGE_CURVE ( 'NONE', #13134, #25424, #205, .T. ) ;
#10180=CARTESIAN_POINT ( 'NONE',  ( 43.81608638205700146, -1.677874310045055051, 19.48083306117937852 ) ) ;
#10181=VECTOR ( 'NONE', #1801, 1000.000000000000000 ) ;
#10184=VECTOR ( 'NONE', #9629, 1000.000000000000114 ) ;
#10197=CARTESIAN_POINT ( 'NONE',  ( 33.31606138205700773, -3.566646240838321269, 18.16837712155798457 ) ) ;
#10213=VERTEX_POINT ( 'NONE', #15806 ) ;
#10219=ORIENTED_EDGE ( 'NONE', *, *, #10364, .F. ) ;
#10224=EDGE_CURVE ( 'NONE', #11138, #19881, #13501, .T. ) ;
#10229=CARTESIAN_POINT ( 'NONE',  ( 32.81606138205700773, -32.95845724189726411, 59.23979596822106686 ) ) ;
#10231=FACE_OUTER_BOUND ( 'NONE', #23991, .T. ) ;
#10232=DIRECTION ( 'NONE',  ( 0.000000000000000000, -0.5706330172266907974, 0.8212051873014217795 ) ) ;
#10236=VECTOR ( 'NONE', #18999, 1000.000000000000000 ) ;
#10237=ORIENTED_EDGE ( 'NONE', *, *, #15077, .F. ) ;
#10244=EDGE_CURVE ( 'NONE', #14645, #2100, #12077, .T. ) ;
#10259=VECTOR ( 'NONE', #20726, 1000.000000000000000 ) ;
#10261=DIRECTION ( 'NONE',  ( 0.000000000000000000, -0.8212051873014252212, -0.5706330172266858014 ) ) ;
#10283=DIRECTION ( 'NONE',  ( -1.000000000000000000, -1.185526135920242153E-16, -8.246758300215675884E-17 ) ) ;
#10314=VERTEX_POINT ( 'NONE', #12967 ) ;
#10327=CARTESIAN_POINT ( 'NONE',  ( 43.11717982288782025, 3.481773294781324690, 6.342591232598341122 ) ) ;
#10342=CIRCLE ( 'NONE', #48, 0.4999999999999943379 ) ;
#10363=FACE_OUTER_BOUND ( 'NONE', #3392, .T. ) ;
#10364=EDGE_CURVE ( 'NONE', #11492, #24026, #10526, .T. ) ;
#10376=ORIENTED_EDGE ( 'NONE', *, *, #13756, .T. ) ;
#10412=AXIS2_PLACEMENT_3D ( 'NONE', #22261, #24058, #6548 ) ;
#10416=CIRCLE ( 'NONE', #513, 0.7500000000000006661 ) ;
#10424=CARTESIAN_POINT ( 'NONE',  ( 33.23058527440272059, 3.113468987225112006, 6.136968036621317069 ) ) ;
#10430=FACE_OUTER_BOUND ( 'NONE', #2886, .T. ) ;
#10436=ORIENTED_EDGE ( 'NONE', *, *, #15933, .F. ) ;
#10438=AXIS2_PLACEMENT_3D ( 'NONE', #12153, #9828, #16112 ) ;
#10442=FACE_OUTER_BOUND ( 'NONE', #14376, .T. ) ;
#10443=CARTESIAN_POINT ( 'NONE',  ( 43.81606138205700063, -33.36905983554797217, 58.95447945960771818 ) ) ;
#10460=FACE_BOUND ( 'NONE', #21013, .T. ) ;
#10500=CARTESIAN_POINT ( 'NONE',  ( 33.33121445922205339, -32.87633672316712108, 59.29685926994373091 ) ) ;
#10515=CIRCLE ( 'NONE', #17097, 0.7499999999999983347 ) ;
#10523=EDGE_CURVE ( 'NONE', #19561, #5208, #9493, .T. ) ;
#10526=LINE ( 'NONE', #24653, #4251 ) ;
#10530=ORIENTED_EDGE ( 'NONE', *, *, #13047, .T. ) ;
#10556=EDGE_CURVE ( 'NONE', #10887, #20815, #17461, .T. ) ;
#10564=EDGE_CURVE ( 'NONE', #4853, #14092, #17328, .T. ) ;
#10570=PLANE ( 'NONE',  #17503 ) ;
#10576=CIRCLE ( 'NONE', #24936, 1.500000000000006217 ) ;
#10588=AXIS2_PLACEMENT_3D ( 'NONE', #3878, #11244, #1433 ) ;
#10610=CARTESIAN_POINT ( 'NONE',  ( 43.79080625344859357, -32.95845724189726411, 59.23979596822106686 ) ) ;
#10611=EDGE_CURVE ( 'NONE', #11314, #6791, #7972, .T. ) ;
#10617=DIRECTION ( 'NONE',  ( 0.000000000000000000, 0.5706330172266920187, -0.8212051873014210024 ) ) ;
#10618=CARTESIAN_POINT ( 'NONE',  ( 32.81606138205700773, 4.124002793203064066, 6.312068993173404863 ) ) ;
#10631=CARTESIAN_POINT ( 'NONE',  ( 42.56606138205700063, 2.740850673309605412, 6.112030963703427133 ) ) ;
#10638=ORIENTED_EDGE ( 'NONE', *, *, #5767, .T. ) ;
#10640=LINE ( 'NONE', #2505, #87 ) ;
#10649=CIRCLE ( 'NONE', #25003, 2.500000000000002220 ) ;
#10655=LINE ( 'NONE', #18503, #23548 ) ;
#10662=CARTESIAN_POINT ( 'NONE',  ( 33.31606138205700773, -36.11063010576116739, 71.66210679335823386 ) ) ;
#10696=ADVANCED_FACE ( 'NONE', ( #10231 ), #21019, .T. ) ;
#10702=VECTOR ( 'NONE', #20060, 1000.000000000000000 ) ;
#10723=DIRECTION ( 'NONE',  ( 0.000000000000000000, 0.5706330172266907974, -0.8212051873014217795 ) ) ;
#10733=CARTESIAN_POINT ( 'NONE',  ( 33.31606138205700773, -35.41471100349711065, 71.53682070832086026 ) ) ;
#10734=DIRECTION ( 'NONE',  ( -1.000000000000000000, 0.000000000000000000, 0.000000000000000000 ) ) ;
#10747=ADVANCED_FACE ( 'NONE', ( #12804 ), #18722, .T. ) ;
#10750=CARTESIAN_POINT ( 'NONE',  ( 33.56477571746443544, 3.418883076854447367, 6.349191931652266696 ) ) ;
#10760=ORIENTED_EDGE ( 'NONE', *, *, #199, .F. ) ;
#10782=EDGE_CURVE ( 'NONE', #6498, #8460, #18268, .T. ) ;
#10787=CARTESIAN_POINT ( 'NONE',  ( 43.69896204258590444, 3.548173818309678484, 6.215045287937394747 ) ) ;
#10799=CARTESIAN_POINT ( 'NONE',  ( 33.23058527440272059, 3.113468987225112006, 6.136968036621317069 ) ) ;
#10800=CARTESIAN_POINT ( 'NONE',  ( 33.24019963865212191, 3.104051971978903701, 6.135536383744724098 ) ) ;
#10822=CARTESIAN_POINT ( 'NONE',  ( 33.31606138205700773, -2.088476903695762665, 19.19551655256602984 ) ) ;
#10844=CIRCLE ( 'NONE', #24393, 0.5000000000000001110 ) ;
#10861=LINE ( 'NONE', #3234, #17023 ) ;
#10874=CARTESIAN_POINT ( 'NONE',  ( 33.57054761034910229, 3.412271088041349820, 6.349711998884802533 ) ) ;
#10887=VERTEX_POINT ( 'NONE', #20270 ) ;
#10888=EDGE_CURVE ( 'NONE', #6498, #22104, #24367, .T. ) ;
#10890=CARTESIAN_POINT ( 'NONE',  ( 43.81606138205700063, 3.913963181809303027, 6.295759124378626836 ) ) ;
#10894=CARTESIAN_POINT ( 'NONE',  ( 43.31606138205700063, -38.37466412126273951, 70.68129701848354784 ) ) ;
#10897=ORIENTED_EDGE ( 'NONE', *, *, #6983, .F. ) ;
#10918=CARTESIAN_POINT ( 'NONE',  ( 34.06606138205700773, -40.62725863591898445, 68.52362519861142687 ) ) ;
#10938=VERTEX_POINT ( 'NONE', #1783 ) ;
#10960=DIRECTION ( 'NONE',  ( -1.000000000000000000, -1.518641380243644581E-16, -1.055262346480601087E-16 ) ) ;
#10969=ADVANCED_FACE ( 'NONE', ( #13185 ), #24875, .T. ) ;
#10971=EDGE_LOOP ( 'NONE', ( #3912, #10436, #23478, #5214 ) ) ;
#11005=CARTESIAN_POINT ( 'NONE',  ( 32.81606138205700773, -27.25871422114667553, 59.79942265548595515 ) ) ;
#11017=CLOSED_SHELL ( 'NONE', ( #20338, #1377, #23533, #6727, #10969, #2684, #9734, #9619, #17436, #19186, #16900, #17073, #19003, #17284, #12114, #13191, #21770, #1525, #2546, #22117, #5174, #12541, #1491, #12268, #12574, #5304, #8235, #3558, #15392, #7556, #8494, #9954, #2163, #4376, #10696, #9034, #12559, #15704, #11399, #15297, #8477, #16224, #7276, #16821, #420, #22963, #11774, #6740, #23807, #15011, #18437, #2544, #8751, #3461, #22288, #11806, #16975, #6578, #22142, #17238, #6426, #22188, #19459, #8942, #9874, #12808, #16226, #252, #17740, #12514, #10747, #11535, #23278, #19179, #13373 ) ) ;
#11018=DIRECTION ( 'NONE',  ( -0.000000000000000000, -0.8212051873014210024, -0.5706330172266920187 ) ) ;
#11026=( LENGTH_UNIT ( ) NAMED_UNIT ( * ) SI_UNIT ( .MILLI., .METRE. ) );
#11066=DIRECTION ( 'NONE',  ( -1.849283715844614702E-16, 0.8212051873014210024, 0.5706330172266920187 ) ) ;
#11069=PRODUCT_DEFINITION_CONTEXT ( 'detailed design', #12622, 'design' ) ;
#11121=B_SPLINE_CURVE_WITH_KNOTS ( 'NONE', 3,
 ( #10631, #18482, #14612, #816 ),
 .UNSPECIFIED., .F., .F.,
 ( 4, 4 ),
 ( 0.000000000000000000, 1.000000000000000000 ),
 .UNSPECIFIED. ) ;
#11138=VERTEX_POINT ( 'NONE', #8236 ) ;
#11146=CYLINDRICAL_SURFACE ( 'NONE', #8367, 0.7499999999999983347 ) ;
#11153=ORIENTED_EDGE ( 'NONE', *, *, #23732, .F. ) ;
#11156=AXIS2_PLACEMENT_3D ( 'NONE', #10180, #4511, #21903 ) ;
#11167=CARTESIAN_POINT ( 'NONE',  ( 43.81606138205700063, -33.60910547091194900, 60.61426200347987248 ) ) ;
#11182=ORIENTED_EDGE ( 'NONE', *, *, #9884, .F. ) ;
#11186=CARTESIAN_POINT ( 'NONE',  ( 42.99498874235398205, 2.839582837266055204, 6.102945014747132468 ) ) ;
#11187=AXIS2_PLACEMENT_3D ( 'NONE', #5191, #5057, #18582 ) ;
#11194=EDGE_CURVE ( 'NONE', #24026, #4345, #14033, .T. ) ;
#11195=LINE ( 'NONE', #9140, #769 ) ;
#11196=DIRECTION ( 'NONE',  ( -1.000000000000000000, 0.000000000000000000, 0.000000000000000000 ) ) ;
#11208=EDGE_CURVE ( 'NONE', #1002, #10213, #18648, .T. ) ;
#11227=ORIENTED_EDGE ( 'NONE', *, *, #5793, .F. ) ;
#11244=DIRECTION ( 'NONE',  ( -0.000000000000000000, -0.8212051873014210024, -0.5706330172266920187 ) ) ;
#11256=ORIENTED_EDGE ( 'NONE', *, *, #25160, .T. ) ;
#11262=CARTESIAN_POINT ( 'NONE',  ( 34.06606138205700773, -32.75315594507191008, 59.38245422252773409 ) ) ;
#11265=VECTOR ( 'NONE', #25028, 1000.000000000000114 ) ;
#11269=B_SPLINE_CURVE_WITH_KNOTS ( 'NONE', 3,
 ( #25031, #5483, #7289, #5358 ),
 .UNSPECIFIED., .F., .F.,
 ( 4, 4 ),
 ( 0.000000000000000000, 1.000000000000000000 ),
 .UNSPECIFIED. ) ;
#11270=B_SPLINE_CURVE_WITH_KNOTS ( 'NONE', 3,
 ( #14909, #18527, #12498, #8617 ),
 .UNSPECIFIED., .F., .F.,
 ( 4, 4 ),
 ( 0.000000000000000000, 1.000000000000000000 ),
 .UNSPECIFIED. ) ;
#11275=DIRECTION ( 'NONE',  ( 1.000000000000000000, 0.000000000000000000, 0.000000000000000000 ) ) ;
#11283=CARTESIAN_POINT ( 'NONE',  ( 43.81606138205700063, 3.913817537272060054, 6.295724427891637554 ) ) ;
#11293=COLOUR_RGB ( '', 0.72549020, 0.75294118, 0.79215686) ;
#11303=CARTESIAN_POINT ( 'NONE',  ( 43.81606138205700063, -33.39268706791821018, 60.15578316240965506 ) ) ;
#11314=VERTEX_POINT ( 'NONE', #22517 ) ;
#11329=DIRECTION ( 'NONE',  ( -1.849283715844614702E-16, 0.8212051873014210024, 0.5706330172266920187 ) ) ;
#11331=CARTESIAN_POINT ( 'NONE',  ( 43.81606138205700063, -35.41471100349711065, 71.53682070832086026 ) ) ;
#11375=CARTESIAN_POINT ( 'NONE',  ( 33.80700582398852561, 3.227014992217426492, 6.369498915812663142 ) ) ;
#11384=EDGE_CURVE ( 'NONE', #5709, #4360, #17113, .T. ) ;
#11393=DIRECTION ( 'NONE',  ( -1.000000000000000000, -1.185941393278724777E-16, -8.240782279085522416E-17 ) ) ;
#11399=ADVANCED_FACE ( 'NONE', ( #7317 ), #16589, .F. ) ;
#11404=DIRECTION ( 'NONE',  ( -1.000000000000000000, 0.000000000000000000, 0.000000000000000000 ) ) ;
#11407=ORIENTED_EDGE ( 'NONE', *, *, #25429, .T. ) ;
#11409=AXIS2_PLACEMENT_3D ( 'NONE', #15748, #23603, #16630 ) ;
#11425=DIRECTION ( 'NONE',  ( -1.849283715844614702E-16, 0.8212051873014210024, 0.5706330172266920187 ) ) ;
#11437=LINE ( 'NONE', #23517, #21483 ) ;
#11451=CYLINDRICAL_SURFACE ( 'NONE', #1136, 2.500000000000002220 ) ;
#11453=EDGE_CURVE ( 'NONE', #17862, #3296, #7615, .T. ) ;
#11454=VERTEX_POINT ( 'NONE', #19547 ) ;
#11457=VERTEX_POINT ( 'NONE', #21612 ) ;
#11492=VERTEX_POINT ( 'NONE', #13252 ) ;
#11496=DIRECTION ( 'NONE',  ( 0.000000000000000000, 0.5706330172266919076, -0.8212051873014208914 ) ) ;
#11502=AXIS2_PLACEMENT_3D ( 'NONE', #21256, #23180, #3352 ) ;
#11504=CARTESIAN_POINT ( 'NONE',  ( 33.77225884907574027, 2.787429531901909119, 6.090838246671958167 ) ) ;
#11535=ADVANCED_FACE ( 'NONE', ( #7831 ), #15426, .F. ) ;
#11540=CARTESIAN_POINT ( 'NONE',  ( 33.97785981915764353, 3.164009542016340770, 6.379277577726464088 ) ) ;
#11544=FILL_AREA_STYLE ('',( #15395 ) ) ;
#11547=AXIS2_PLACEMENT_3D ( 'NONE', #5428, #21147, #19844 ) ;
#11552=CARTESIAN_POINT ( 'NONE',  ( 36.56606138205700063, 5.719301844480432884, 2.701924129460374413 ) ) ;
#11556=ORIENTED_EDGE ( 'NONE', *, *, #16105, .F. ) ;
#11564=CARTESIAN_POINT ( 'NONE',  ( 33.33121445922205339, -32.87633672316712108, 59.29685926994373091 ) ) ;
#11575=CARTESIAN_POINT ( 'NONE',  ( 43.05893253799203535, 3.408563886989315339, 6.350990360017436664 ) ) ;
#11618=EDGE_CURVE ( 'NONE', #1658, #3066, #16184, .T. ) ;
#11640=CARTESIAN_POINT ( 'NONE',  ( 33.49067756756858927, 3.520309816310820406, 6.331808112780875852 ) ) ;
#11656=ORIENTED_EDGE ( 'NONE', *, *, #10556, .F. ) ;
#11670=DIRECTION ( 'NONE',  ( -3.771137991253929559E-16, 0.8212051873014208914, 0.5706330172266919076 ) ) ;
#11674=( NAMED_UNIT ( * ) SI_UNIT ( $, .STERADIAN. ) SOLID_ANGLE_UNIT ( ) );
#11700=CARTESIAN_POINT ( 'NONE',  ( 42.99533163877982389, 2.835194748544836330, 6.100154062548608813 ) ) ;
#11733=CARTESIAN_POINT ( 'NONE',  ( 43.31606138205700063, -37.53049398575952722, 70.06662099985003067 ) ) ;
#11738=LINE ( 'NONE', #5795, #4886 ) ;
#11761=CARTESIAN_POINT ( 'NONE',  ( 43.81606138205700063, -35.82531359714782582, 71.25150419970752580 ) ) ;
#11768=EDGE_CURVE ( 'NONE', #17862, #6624, #10655, .T. ) ;
#11774=ADVANCED_FACE ( 'NONE', ( #965 ), #14879, .T. ) ;
#11794=EDGE_LOOP ( 'NONE', ( #20504, #22652, #56, #10154 ) ) ;
#11806=ADVANCED_FACE ( 'NONE', ( #22489 ), #12971, .T. ) ;
#11815=ORIENTED_EDGE ( 'NONE', *, *, #12407, .F. ) ;
#11835=CARTESIAN_POINT ( 'NONE',  ( 43.31606138205700063, -35.70002751211045933, 71.94742330197156832 ) ) ;
#11838=AXIS2_PLACEMENT_3D ( 'NONE', #15606, #1816, #7383 ) ;
#11843=ORIENTED_EDGE ( 'NONE', *, *, #15075, .T. ) ;
#11866=EDGE_LOOP ( 'NONE', ( #24262, #18076, #21530, #20066 ) ) ;
#11870=ORIENTED_EDGE ( 'NONE', *, *, #7346, .T. ) ;
#11874=VECTOR ( 'NONE', #22521, 1000.000000000000114 ) ;
#11884=B_SPLINE_CURVE_WITH_KNOTS ( 'NONE', 3,
 ( #16353, #14058, #14436, #19854 ),
 .UNSPECIFIED., .F., .F.,
 ( 4, 4 ),
 ( 0.000000000000000000, 0.9997489389489839784 ),
 .UNSPECIFIED. ) ;
#11894=CARTESIAN_POINT ( 'NONE',  ( 33.31606138205700773, 3.172506336381830661, 12.50058896911730066 ) ) ;
#11906=VECTOR ( 'NONE', #7003, 1000.000000000000114 ) ;
#11915=PRESENTATION_STYLE_ASSIGNMENT (( #1967 ) ) ;
#11920=ORIENTED_EDGE ( 'NONE', *, *, #21669, .F. ) ;
#11922=CARTESIAN_POINT ( 'NONE',  ( 43.31606138205700063, 7.166937456968672571, 6.752152658007350539 ) ) ;
#11926=CIRCLE ( 'NONE', #17248, 2.500000000000002220 ) ;
#11933=CIRCLE ( 'NONE', #18928, 0.5000000000000008882 ) ;
#11989=LINE ( 'NONE', #19954, #4629 ) ;
#11992=VECTOR ( 'NONE', #21720, 1000.000000000000114 ) ;
#12004=B_SPLINE_SURFACE_WITH_KNOTS ( 'NONE', 1, 3, ( 
 ( #14413, #14539, #20848, #4748 ),
 ( #7063, #24178, #8749, #12623 ),
 ( #998, #12751, #14656, #6552 ) ),
 .UNSPECIFIED., .F., .F., .F.,
 ( 2, 1, 2 ),
 ( 4, 4 ),
 ( -0.01000000000000000021, 0.000000000000000000, 1.000000000000000000 ),
 ( 0.000000000000000000, 1.000000000000000000 ),
 .UNSPECIFIED. ) ;
#12015=DIRECTION ( 'NONE',  ( 0.000000000000000000, 0.5706330172266930179, -0.8212051873014202252 ) ) ;
#12069=EDGE_LOOP ( 'NONE', ( #14502, #5879, #13235, #702 ) ) ;
#12074=CARTESIAN_POINT ( 'NONE',  ( 40.56606138205700773, 6.004618353093779781, 2.291321535809666354 ) ) ;
#12076=CARTESIAN_POINT ( 'NONE',  ( 42.56606138205700063, -40.62725863591898445, 68.52362519861142687 ) ) ;
#12077=CIRCLE ( 'NONE', #933, 0.7500000000000031086 ) ;
#12080=ORIENTED_EDGE ( 'NONE', *, *, #6413, .T. ) ;
#12096=VECTOR ( 'NONE', #18344, 1000.000000000000000 ) ;
#12099=EDGE_CURVE ( 'NONE', #5726, #13134, #19257, .T. ) ;
#12100=VERTEX_POINT ( 'NONE', #17087 ) ;
#12101=CARTESIAN_POINT ( 'NONE',  ( 43.31606138205700063, -27.17722769842920272, 59.42551550655435477 ) ) ;
#12109=ORIENTED_EDGE ( 'NONE', *, *, #4387, .T. ) ;
#12112=EDGE_CURVE ( 'NONE', #19940, #4607, #11269, .T. ) ;
#12114=ADVANCED_FACE ( 'NONE', ( #25292 ), #15266, .F. ) ;
#12116=CYLINDRICAL_SURFACE ( 'NONE', #25180, 0.4999999999999982792 ) ;
#12119=CARTESIAN_POINT ( 'NONE',  ( 33.39768049593357091, 3.266176032039786570, 6.243079984136794991 ) ) ;
#12144=CARTESIAN_POINT ( 'NONE',  ( 33.31606138205700773, -0.3976309214372003575, 10.62865949386124242 ) ) ;
#12150=DIRECTION ( 'NONE',  ( 1.000000000000000000, 5.723954245484026287E-31, -8.237414899530862620E-31 ) ) ;
#12153=CARTESIAN_POINT ( 'NONE',  ( 43.81608638205700146, -3.566646240838321269, 18.16837712155798457 ) ) ;
#12172=CYLINDRICAL_SURFACE ( 'NONE', #9263, 0.5000000000000004441 ) ;
#12177=VERTEX_POINT ( 'NONE', #4051 ) ;
#12180=DIRECTION ( 'NONE',  ( -1.000000000000000000, 0.000000000000000000, 0.000000000000000000 ) ) ;
#12183=ORIENTED_EDGE ( 'NONE', *, *, #7346, .F. ) ;
#12207=ORIENTED_EDGE ( 'NONE', *, *, #13592, .T. ) ;
#12229=CARTESIAN_POINT ( 'NONE',  ( 43.14003743237937982, 2.901513403460370455, 6.097021259270054117 ) ) ;
#12230=DIRECTION ( 'NONE',  ( 0.000000000000000000, -0.5706330172266919076, 0.8212051873014208914 ) ) ;
#12247=ORIENTED_EDGE ( 'NONE', *, *, #17948, .T. ) ;
#12253=CIRCLE ( 'NONE', #7726, 0.4999999999999994449 ) ;
#12263=CARTESIAN_POINT ( 'NONE',  ( 43.81606138205700063, 4.103895195095678794, 6.341006091748962348 ) ) ;
#12265=DIRECTION ( 'NONE',  ( -1.000000000000000000, -7.497642437004238434E-16, 3.111695294957277996E-17 ) ) ;
#12268=ADVANCED_FACE ( 'NONE', ( #18349 ), #24372, .F. ) ;
#12270=DIRECTION ( 'NONE',  ( 0.000000000000000000, -0.5706330172266915746, 0.8212051873014213355 ) ) ;
#12282=EDGE_LOOP ( 'NONE', ( #20827, #13820, #12679, #19760 ) ) ;
#12284=ORIENTED_EDGE ( 'NONE', *, *, #10523, .F. ) ;
#12288=ORIENTED_EDGE ( 'NONE', *, *, #20302, .T. ) ;
#12290=ORIENTED_EDGE ( 'NONE', *, *, #19252, .F. ) ;
#12301=CARTESIAN_POINT ( 'NONE',  ( 33.80700582398836218, 3.227014992217502876, 6.369498915812659590 ) ) ;
#12312=VECTOR ( 'NONE', #24373, 1000.000000000000114 ) ;
#12314=ORIENTED_EDGE ( 'NONE', *, *, #3445, .T. ) ;
#12333=ORIENTED_EDGE ( 'NONE', *, *, #11768, .F. ) ;
#12334=ORIENTED_EDGE ( 'NONE', *, *, #10556, .T. ) ;
#12337=CARTESIAN_POINT ( 'NONE',  ( 43.05893433410182070, 3.408565912792066221, 6.350990188909392486 ) ) ;
#12350=ORIENTED_EDGE ( 'NONE', *, *, #14939, .T. ) ;
#12362=FACE_OUTER_BOUND ( 'NONE', #6555, .T. ) ;
#12365=DIRECTION ( 'NONE',  ( 0.000000000000000000, 0.5706330172266919076, -0.8212051873014208914 ) ) ;
#12367=EDGE_CURVE ( 'NONE', #20521, #13577, #23570, .T. ) ;
#12387=CARTESIAN_POINT ( 'NONE',  ( 43.39709375099405975, 3.108381023609500193, 6.137326095127844994 ) ) ;
#12402=DIRECTION ( 'NONE',  ( -1.000000000000000000, 0.000000000000000000, 0.000000000000000000 ) ) ;
#12403=EDGE_LOOP ( 'NONE', ( #5421, #9317, #13949, #6313 ) ) ;
#12407=EDGE_CURVE ( 'NONE', #17256, #3766, #788, .T. ) ;
#12428=DIRECTION ( 'NONE',  ( 0.000000000000000000, -0.4278636397681519488, 0.9038432971286277651 ) ) ;
#12438=LINE ( 'NONE', #16273, #12312 ) ;
#12453=EDGE_LOOP ( 'NONE', ( #11227, #12480, #19812, #25049, #16286, #12284, #2493, #11815 ) ) ;
#12456=EDGE_LOOP ( 'NONE', ( #3338, #18464, #16098, #15751 ) ) ;
#12462=CIRCLE ( 'NONE', #8333, 0.4999999999999998890 ) ;
#12464=ORIENTED_EDGE ( 'NONE', *, *, #17948, .F. ) ;
#12466=VERTEX_POINT ( 'NONE', #19476 ) ;
#12473=EDGE_CURVE ( 'NONE', #24159, #24513, #25258, .T. ) ;
#12474=EDGE_CURVE ( 'NONE', #10887, #24226, #4654, .T. ) ;
#12476=CARTESIAN_POINT ( 'NONE',  ( 40.81606138205700773, -6.959910619544160681, 20.07251914782758107 ) ) ;
#12480=ORIENTED_EDGE ( 'NONE', *, *, #8021, .F. ) ;
#12495=DIRECTION ( 'NONE',  ( 1.000000000000000000, 0.000000000000000000, 0.000000000000000000 ) ) ;
#12498=CARTESIAN_POINT ( 'NONE',  ( 33.91911362184673351, 2.753402311566605309, 6.093967742448072933 ) ) ;
#12500=CARTESIAN_POINT ( 'NONE',  ( 43.26087622013976386, 3.761531814868369406, 6.334937692063231651 ) ) ;
#12505=DIRECTION ( 'NONE',  ( 1.445602896647339656E-16, -0.8212051873014208914, -0.5706330172266919076 ) ) ;
#12508=B_SPLINE_CURVE_WITH_KNOTS ( 'NONE', 3,
 ( #1100, #19150, #3432, #10787 ),
 .UNSPECIFIED., .F., .F.,
 ( 4, 4 ),
 ( 0.000000000000000000, 1.000000000000000000 ),
 .UNSPECIFIED. ) ;
#12514=ADVANCED_FACE ( 'NONE', ( #19353 ), #13435, .T. ) ;
#12521=FACE_OUTER_BOUND ( 'NONE', #17460, .T. ) ;
#12536=DIRECTION ( 'NONE',  ( -1.734723475976804876E-16, 0.8212051873014210024, 0.5706330172266920187 ) ) ;
#12541=ADVANCED_FACE ( 'NONE', ( #9207 ), #7388, .F. ) ;
#12545=EDGE_LOOP ( 'NONE', ( #16687, #5458 ) ) ;
#12547=CARTESIAN_POINT ( 'NONE',  ( 42.56606138205700063, 3.151453266960317023, 6.397347472316774031 ) ) ;
#12559=ADVANCED_FACE ( 'NONE', ( #21041 ), #17118, .T. ) ;
#12574=ADVANCED_FACE ( 'NONE', ( #21796 ), #23838, .F. ) ;
#12600=CARTESIAN_POINT ( 'NONE',  ( 43.27195111268100192, 2.993280262538516201, 6.111616072109399944 ) ) ;
#12622=APPLICATION_CONTEXT ( 'automotive_design' ) ;
#12623=CARTESIAN_POINT ( 'NONE',  ( 43.69896204258590444, 3.548173818309682037, 6.215045287937394747 ) ) ;
#12658=LINE ( 'NONE', #18326, #2335 ) ;
#12668=CARTESIAN_POINT ( 'NONE',  ( 43.81606138205700063, -3.566646240838321269, 18.16837712155798457 ) ) ;
#12674=FACE_OUTER_BOUND ( 'NONE', #12453, .T. ) ;
#12679=ORIENTED_EDGE ( 'NONE', *, *, #4994, .T. ) ;
#12681=CARTESIAN_POINT ( 'NONE',  ( 32.81606138205700773, -35.41471100349711065, 71.53682070832086026 ) ) ;
#12682=CARTESIAN_POINT ( 'NONE',  ( 32.81606138205700773, -37.34243788671330577, 70.80615726751818784 ) ) ;
#12696=VECTOR ( 'NONE', #22623, 1000.000000000000114 ) ;
#12714=EDGE_CURVE ( 'NONE', #59, #1002, #7573, .T. ) ;
#12717=DIRECTION ( 'NONE',  ( 0.000000000000000000, 0.5706330172266919076, -0.8212051873014208914 ) ) ;
#12750=CIRCLE ( 'NONE', #23424, 2.500000000000002220 ) ;
#12751=CARTESIAN_POINT ( 'NONE',  ( 43.14077072142541169, 3.506326161111083195, 6.337847826736607182 ) ) ;
#12752=CARTESIAN_POINT ( 'NONE',  ( 43.31606138205700063, 6.289375473607850431, 7.138843309009015314 ) ) ;
#12753=DIRECTION ( 'NONE',  ( 0.000000000000000000, 0.5706330172266919076, -0.8212051873014208914 ) ) ;
#12766=DIRECTION ( 'NONE',  ( 0.000000000000000000, 0.000000000000000000, 1.000000000000000000 ) ) ;
#12768=LINE ( 'NONE', #2942, #1447 ) ;
#12773=LINE ( 'NONE', #16743, #4209 ) ;
#12804=FACE_OUTER_BOUND ( 'NONE', #5418, .T. ) ;
#12808=ADVANCED_FACE ( 'NONE', ( #10460, #3090, #1025 ), #8909, .T. ) ;
#12824=ORIENTED_EDGE ( 'NONE', *, *, #24180, .F. ) ;
#12847=ORIENTED_EDGE ( 'NONE', *, *, #10782, .T. ) ;
#12849=DIRECTION ( 'NONE',  ( 0.000000000000000000, -0.8212051873014213355, -0.5706330172266915746 ) ) ;
#12863=DIRECTION ( 'NONE',  ( 0.000000000000000000, -0.8212051873014288850, -0.5706330172266804723 ) ) ;
#12869=CARTESIAN_POINT ( 'NONE',  ( 33.31606138205700773, -10.80800258567212602, 32.62011605800211811 ) ) ;
#12894=ORIENTED_EDGE ( 'NONE', *, *, #3718, .T. ) ;
#12941=AXIS2_PLACEMENT_3D ( 'NONE', #8079, #4083, #13749 ) ;
#12944=VECTOR ( 'NONE', #13340, 1000.000000000000114 ) ;
#12955=LINE ( 'NONE', #14741, #5041 ) ;
#12961=CARTESIAN_POINT ( 'NONE',  ( 43.81606138205700063, -37.34243788671330577, 70.80615726751818784 ) ) ;
#12967=CARTESIAN_POINT ( 'NONE',  ( 43.81606138205700063, 3.172506336381830661, 12.50058896911730066 ) ) ;
#12971=PLANE ( 'NONE',  #16156 ) ;
#12972=ORIENTED_EDGE ( 'NONE', *, *, #17591, .F. ) ;
#12993=LINE ( 'NONE', #16849, #8217 ) ;
#12994=ORIENTED_EDGE ( 'NONE', *, *, #16974, .T. ) ;
#13004=CARTESIAN_POINT ( 'NONE',  ( 36.56606138205700063, 6.004618353093779781, 2.291321535809666354 ) ) ;
#13015=EDGE_LOOP ( 'NONE', ( #5099, #3924 ) ) ;
#13033=VERTEX_POINT ( 'NONE', #24850 ) ;
#13041=ORIENTED_EDGE ( 'NONE', *, *, #19626, .T. ) ;
#13047=EDGE_CURVE ( 'NONE', #11457, #16794, #2295, .T. ) ;
#13055=FACE_OUTER_BOUND ( 'NONE', #14998, .T. ) ;
#13061=CARTESIAN_POINT ( 'NONE',  ( 33.22724336997212902, 3.110414846328807936, 6.134845797670998913 ) ) ;
#13075=EDGE_LOOP ( 'NONE', ( #42, #20330, #1067, #8804 ) ) ;
#13078=CARTESIAN_POINT ( 'NONE',  ( 43.31606138205700063, 4.103895195095678794, 6.341006091748962348 ) ) ;
#13096=CIRCLE ( 'NONE', #1964, 0.5000000000000019984 ) ;
#13110=DIRECTION ( 'NONE',  ( 1.022195611122249672E-16, -0.1771812806364704007, -0.9841782327363373106 ) ) ;
#13112=ORIENTED_EDGE ( 'NONE', *, *, #23432, .F. ) ;
#13121=DIRECTION ( 'NONE',  ( 0.000000000000000000, 0.5706330172266920187, -0.8212051873014210024 ) ) ;
#13122=LINE ( 'NONE', #24816, #15107 ) ;
#13126=EDGE_CURVE ( 'NONE', #19881, #59, #9588, .T. ) ;
#13128=CARTESIAN_POINT ( 'NONE',  ( 43.31606138205700063, -35.70002751211045933, 71.94742330197156832 ) ) ;
#13134=VERTEX_POINT ( 'NONE', #23560 ) ;
#13146=AXIS2_PLACEMENT_3D ( 'NONE', #18293, #16331, #14415 ) ;
#13172=EDGE_LOOP ( 'NONE', ( #13112, #21475, #2387, #19418 ) ) ;
#13183=AXIS2_PLACEMENT_3D ( 'NONE', #23439, #25095, #15838 ) ;
#13185=FACE_OUTER_BOUND ( 'NONE', #22784, .T. ) ;
#13188=CARTESIAN_POINT ( 'NONE',  ( 33.33836326447716658, 3.869514117107255569, 6.310928887378282504 ) ) ;
#13191=ADVANCED_FACE ( 'NONE', ( #7995 ), #15708, .F. ) ;
#13196=EDGE_CURVE ( 'NONE', #59, #6765, #8979, .T. ) ;
#13215=LINE ( 'NONE', #22608, #12944 ) ;
#13216=B_SPLINE_SURFACE_WITH_KNOTS ( 'NONE', 1, 3, ( 
 ( #11167, #11303, #1855, #1480 ),
 ( #13230, #7424, #23369, #7293 ) ),
 .UNSPECIFIED., .F., .F., .F.,
 ( 2, 2 ),
 ( 4, 4 ),
 ( 0.000000000000000000, 1.000000000000000000 ),
 ( 0.000000000000000000, 1.000000000000000000 ),
 .UNSPECIFIED. ) ;
#13230=CARTESIAN_POINT ( 'NONE',  ( 43.31606138205700063, -33.60910547091194900, 60.61426200347987248 ) ) ;
#13235=ORIENTED_EDGE ( 'NONE', *, *, #1042, .F. ) ;
#13238=DIRECTION ( 'NONE',  ( -0.3454074107579455100, -0.7706623348594876521, -0.5355121718713914403 ) ) ;
#13246=AXIS2_PLACEMENT_3D ( 'NONE', #2507, #16682, #16543 ) ;
#13252=CARTESIAN_POINT ( 'NONE',  ( 36.56606138205700063, 5.594015759443068170, 2.006005027196319901 ) ) ;
#13254=DIRECTION ( 'NONE',  ( 1.000000000000000000, -0.000000000000000000, 0.000000000000000000 ) ) ;
#13276=CARTESIAN_POINT ( 'NONE',  ( 43.81606138205700063, -33.36905983554797217, 58.95447945960771818 ) ) ;
#13293=CIRCLE ( 'NONE', #2989, 0.4999999999999998890 ) ;
#13300=ORIENTED_EDGE ( 'NONE', *, *, #10611, .F. ) ;
#13315=SHAPE_DEFINITION_REPRESENTATION ( #15886, #14587 ) ;
#13316=CARTESIAN_POINT ( 'NONE',  ( 33.32111138205700485, 3.997296121548431724, 6.311886478796241207 ) ) ;
#13318=B_SPLINE_CURVE_WITH_KNOTS ( 'NONE', 3,
 ( #22743, #20822, #12600, #2651 ),
 .UNSPECIFIED., .F., .F.,
 ( 4, 4 ),
 ( 0.000000000000000000, 1.000000000000000000 ),
 .UNSPECIFIED. ) ;
#13320=AXIS2_PLACEMENT_3D ( 'NONE', #14594, #8429, #18588 ) ;
#13332=ORIENTED_EDGE ( 'NONE', *, *, #21436, .T. ) ;
#13340=DIRECTION ( 'NONE',  ( 0.000000000000000000, -0.8212051873014208914, -0.5706330172266919076 ) ) ;
#13352=DIRECTION ( 'NONE',  ( -1.000000000000000000, 0.000000000000000000, 0.000000000000000000 ) ) ;
#13367=EDGE_LOOP ( 'NONE', ( #21050, #13472, #9126, #3419 ) ) ;
#13373=ADVANCED_FACE ( 'NONE', ( #24232 ), #16516, .F. ) ;
#13374=CARTESIAN_POINT ( 'NONE',  ( 42.71157262388818054, 2.752950597436833124, 6.094617809961420996 ) ) ;
#13377=ORIENTED_EDGE ( 'NONE', *, *, #23432, .T. ) ;
#13378=EDGE_CURVE ( 'NONE', #24541, #22414, #794, .T. ) ;
#13381=CARTESIAN_POINT ( 'NONE',  ( 43.06277335143801821, 3.412913593199472295, 6.350629247954049816 ) ) ;
#13385=CYLINDRICAL_SURFACE ( 'NONE', #21736, 0.5000000000000008882 ) ;
#13403=DIRECTION ( 'NONE',  ( -1.000000000000000000, -1.187136597504755470E-16, -8.249087426255173666E-17 ) ) ;
#13415=B_SPLINE_SURFACE_WITH_KNOTS ( 'NONE', 1, 3, ( 
 ( #140, #9949, #1680, #1938 ),
 ( #3620, #11504, #23457, #7634 ),
 ( #11375, #13681, #25377, #5823 ) ),
 .UNSPECIFIED., .F., .F., .F.,
 ( 2, 1, 2 ),
 ( 4, 4 ),
 ( -0.01000000000000000021, 0.000000000000000000, 1.000000000000000000 ),
 ( 0.000000000000000000, 1.000000000000000000 ),
 .UNSPECIFIED. ) ;
#13435=PLANE ( 'NONE',  #19888 ) ;
#13445=CARTESIAN_POINT ( 'NONE',  ( 32.81606138205700773, -1.963190818658398173, 19.89143565483009013 ) ) ;
#13472=ORIENTED_EDGE ( 'NONE', *, *, #3578, .T. ) ;
#13489=CARTESIAN_POINT ( 'NONE',  ( 42.99635608599476200, 2.840112565366839092, 6.103054897711724713 ) ) ;
#13490=EDGE_CURVE ( 'NONE', #4607, #3296, #10013, .T. ) ;
#13498=VECTOR ( 'NONE', #10143, 1000.000000000000114 ) ;
#13501=B_SPLINE_CURVE_WITH_KNOTS ( 'NONE', 3,
 ( #326, #14006, #14258, #12337 ),
 .UNSPECIFIED., .F., .F.,
 ( 4, 4 ),
 ( 0.000000000000000000, 1.000000000000000000 ),
 .UNSPECIFIED. ) ;
#13518=CARTESIAN_POINT ( 'NONE',  ( 43.31606138205700063, 2.761903742731119049, 12.21527246050395377 ) ) ;
#13523=DIRECTION ( 'NONE',  ( 0.000000000000000000, -0.5706330172266952383, 0.8212051873014186709 ) ) ;
#13524=DIRECTION ( 'NONE',  ( 1.000000000000000000, 1.518641380243644581E-16, 1.055262346480601087E-16 ) ) ;
#13530=AXIS2_PLACEMENT_3D ( 'NONE', #15485, #3253, #15234 ) ;
#13534=ORIENTED_EDGE ( 'NONE', *, *, #8621, .F. ) ;
#13553=FACE_BOUND ( 'NONE', #20866, .T. ) ;
#13556=CARTESIAN_POINT ( 'NONE',  ( 43.31606138205700063, 4.529600202371326212, 14.05245759722139454 ) ) ;
#13561=CARTESIAN_POINT ( 'NONE',  ( 33.56477571746444255, 3.418883076854433600, 6.349191931652259591 ) ) ;
#13577=VERTEX_POINT ( 'NONE', #14488 ) ;
#13592=EDGE_CURVE ( 'NONE', #16794, #4227, #16157, .T. ) ;
#13605=VERTEX_POINT ( 'NONE', #2498 ) ;
#13662=CARTESIAN_POINT ( 'NONE',  ( 32.81606138205700773, 3.172506336381830661, 12.50058896911730066 ) ) ;
#13674=CARTESIAN_POINT ( 'NONE',  ( 32.81606138205700773, -40.62725863591898445, 68.52362519861142687 ) ) ;
#13675=CARTESIAN_POINT ( 'NONE',  ( 43.81606138205700063, 4.529600202371326212, 14.05245759722139454 ) ) ;
#13681=CARTESIAN_POINT ( 'NONE',  ( 33.88977883057645357, 3.189440312111338383, 6.370184205214554751 ) ) ;
#13691=VECTOR ( 'NONE', #15664, 1000.000000000000000 ) ;
#13697=ORIENTED_EDGE ( 'NONE', *, *, #23591, .T. ) ;
#13705=VERTEX_POINT ( 'NONE', #24887 ) ;
#13714=VECTOR ( 'NONE', #4036, 1000.000000000000000 ) ;
#13717=EDGE_LOOP ( 'NONE', ( #15328, #6185, #20495, #14525 ) ) ;
#13730=AXIS2_PLACEMENT_3D ( 'NONE', #3109, #9064, #18832 ) ;
#13734=LINE ( 'NONE', #7430, #10184 ) ;
#13749=DIRECTION ( 'NONE',  ( -1.000000000000000000, 0.000000000000000000, 0.000000000000000000 ) ) ;
#13756=EDGE_CURVE ( 'NONE', #22006, #1510, #6357, .T. ) ;
#13757=AXIS2_PLACEMENT_3D ( 'NONE', #12961, #11018, #11404 ) ;
#13775=LINE ( 'NONE', #9667, #25305 ) ;
#13799=CARTESIAN_POINT ( 'NONE',  ( 43.81606138205700063, -37.98241563432385703, 69.85268917996594951 ) ) ;
#13800=LINE ( 'NONE', #13675, #18265 ) ;
#13810=CARTESIAN_POINT ( 'NONE',  ( 43.06468080341912241, 3.415100481987967562, 6.350457055188933886 ) ) ;
#13820=ORIENTED_EDGE ( 'NONE', *, *, #25301, .T. ) ;
#13842=CARTESIAN_POINT ( 'NONE',  ( 35.81606138205700063, -6.959910619544162458, 20.07251914782757751 ) ) ;
#13855=ORIENTED_EDGE ( 'NONE', *, *, #4387, .F. ) ;
#13862=DIRECTION ( 'NONE',  ( 1.000000000000000000, 0.000000000000000000, 0.000000000000000000 ) ) ;
#13873=ORIENTED_EDGE ( 'NONE', *, *, #11194, .T. ) ;
#13889=ORIENTED_EDGE ( 'NONE', *, *, #8021, .T. ) ;
#13896=DIRECTION ( 'NONE',  ( 0.000000000000000000, -0.9841782327363374216, 0.1771812806364704285 ) ) ;
#13932=DIRECTION ( 'NONE',  ( -1.000000000000000000, 0.000000000000000000, 0.000000000000000000 ) ) ;
#13943=DIRECTION ( 'NONE',  ( -1.000000000000000000, -6.197457809535974789E-17, -1.134781633102316229E-16 ) ) ;
#13949=ORIENTED_EDGE ( 'NONE', *, *, #2650, .F. ) ;
#13960=CARTESIAN_POINT ( 'NONE',  ( 43.81606138205700063, -20.88462213363798270, 44.49284693533410717 ) ) ;
#13974=EDGE_CURVE ( 'NONE', #6791, #9087, #9466, .T. ) ;
#13976=VERTEX_POINT ( 'NONE', #3519 ) ;
#13979=ORIENTED_EDGE ( 'NONE', *, *, #7364, .F. ) ;
#13983=VERTEX_POINT ( 'NONE', #15493 ) ;
#13989=DIRECTION ( 'NONE',  ( 0.000000000000000000, 0.8212051873014208914, 0.5706330172266919076 ) ) ;
#14006=CARTESIAN_POINT ( 'NONE',  ( 42.90907157547734840, 3.273800194541344855, 6.355715097684958792 ) ) ;
#14009=LINE ( 'NONE', #21862, #13498 ) ;
#14014=CARTESIAN_POINT ( 'NONE',  ( 38.31606138205700063, -29.37462871496113337, 53.20604314849776983 ) ) ;
#14020=CARTESIAN_POINT ( 'NONE',  ( 33.31606138205700773, -39.23120981750657421, 69.49370132789680099 ) ) ;
#14028=CARTESIAN_POINT ( 'NONE',  ( 40.56606138205700773, 5.594015759443068170, 2.006005027196319901 ) ) ;
#14033=LINE ( 'NONE', #17909, #15317 ) ;
#14055=DIRECTION ( 'NONE',  ( 0.000000000000000000, -0.5706330172266896872, 0.8212051873014225567 ) ) ;
#14058=CARTESIAN_POINT ( 'NONE',  ( 33.23377536606392368, 3.110316458148107976, 6.136481421541682302 ) ) ;
#14077=ORIENTED_EDGE ( 'NONE', *, *, #19086, .T. ) ;
#14088=LINE ( 'NONE', #23987, #4305 ) ;
#14092=VERTEX_POINT ( 'NONE', #21808 ) ;
#14100=EDGE_LOOP ( 'NONE', ( #23407, #11256, #21513, #1459 ) ) ;
#14107=EDGE_LOOP ( 'NONE', ( #1614, #17344, #18571, #8699 ) ) ;
#14118=ORIENTED_EDGE ( 'NONE', *, *, #13126, .F. ) ;
#14120=DIRECTION ( 'NONE',  ( 1.000000000000000000, 1.288820809889844211E-16, 6.101052743105423043E-17 ) ) ;
#14127=DIRECTION ( 'NONE',  ( 0.000000000000000000, 0.5706330172266919076, -0.8212051873014208914 ) ) ;
#14142=DIRECTION ( 'NONE',  ( -1.734723475976804876E-16, 0.8212051873014210024, 0.5706330172266920187 ) ) ;
#14160=DIRECTION ( 'NONE',  ( -1.000000000000000000, 0.000000000000000000, 0.000000000000000000 ) ) ;
#14163=CARTESIAN_POINT ( 'NONE',  ( 43.05893253799167297, 3.408563886988916103, 6.350990360017464198 ) ) ;
#14171=DIRECTION ( 'NONE',  ( 1.000000000000000000, -0.000000000000000000, 0.000000000000000000 ) ) ;
#14178=PLANE ( 'NONE',  #14818 ) ;
#14201=CARTESIAN_POINT ( 'NONE',  ( 43.09178375111335413, 3.447594731875835983, 6.345965694596597650 ) ) ;
#14223=CARTESIAN_POINT ( 'NONE',  ( 32.81606138205700773, -33.60910547091194900, 60.61426200347987248 ) ) ;
#14232=EDGE_CURVE ( 'NONE', #19839, #11138, #295, .T. ) ;
#14238=LINE ( 'NONE', #22082, #24700 ) ;
#14251=DIRECTION ( 'NONE',  ( -1.000000000000000000, -1.185941393278724777E-16, -8.240782279085522416E-17 ) ) ;
#14253=CARTESIAN_POINT ( 'NONE',  ( 43.81606138205700063, -20.45664737071796324, 43.87694304485803798 ) ) ;
#14258=CARTESIAN_POINT ( 'NONE',  ( 42.98956905832363873, 3.335839619496017594, 6.349669990344222192 ) ) ;
#14277=CARTESIAN_POINT ( 'NONE',  ( 43.27190301404667849, 2.993235644242374871, 6.111605774860289664 ) ) ;
#14304=CARTESIAN_POINT ( 'NONE',  ( 32.81606138205700773, -27.17722769842920272, 59.42551550655435477 ) ) ;
#14310=CARTESIAN_POINT ( 'NONE',  ( 43.31606138205700063, -34.55876147765707174, 70.30501292736873609 ) ) ;
#14338=CARTESIAN_POINT ( 'NONE',  ( 32.84131651066541480, -32.95845724189726411, 59.23979596822106686 ) ) ;
#14354=DIRECTION ( 'NONE',  ( -1.000000000000000000, 0.000000000000000000, 0.000000000000000000 ) ) ;
#14356=CARTESIAN_POINT ( 'NONE',  ( 43.22322292330370175, 3.253818082689177160, 6.243461734314118772 ) ) ;
#14364=AXIS2_PLACEMENT_3D ( 'NONE', #10168, #8111, #17913 ) ;
#14376=EDGE_LOOP ( 'NONE', ( #20027, #9941, #9306, #2773 ) ) ;
#14383=CARTESIAN_POINT ( 'NONE',  ( 43.81608638205700146, 0.9984178969752143251, 11.59873562314662010 ) ) ;
#14407=CARTESIAN_POINT ( 'NONE',  ( 40.06606138205700063, 5.308699250829721272, 2.416607620847027960 ) ) ;
#14413=CARTESIAN_POINT ( 'NONE',  ( 43.40041788046962523, 3.105313829025544425, 6.135194785527184891 ) ) ;
#14415=DIRECTION ( 'NONE',  ( 1.000000000000000000, 0.000000000000000000, 0.000000000000000000 ) ) ;
#14431=DIRECTION ( 'NONE',  ( 0.000000000000000000, 0.5706330172266920187, -0.8212051873014210024 ) ) ;
#14436=CARTESIAN_POINT ( 'NONE',  ( 33.23698021073552411, 3.107177411735388084, 6.136004175196663191 ) ) ;
#14456=CARTESIAN_POINT ( 'NONE',  ( 42.82259739205072435, 3.224889171211050343, 6.370942055173422602 ) ) ;
#14488=CARTESIAN_POINT ( 'NONE',  ( 33.31606138205700773, 2.476587234117772596, 12.62587505415466538 ) ) ;
#14502=ORIENTED_EDGE ( 'NONE', *, *, #3158, .T. ) ;
#14509=CARTESIAN_POINT ( 'NONE',  ( 32.81606138205700773, -35.70002751211045933, 71.94742330197156832 ) ) ;
#14525=ORIENTED_EDGE ( 'NONE', *, *, #25160, .F. ) ;
#14535=CYLINDRICAL_SURFACE ( 'NONE', #8356, 1.250000000000001110 ) ;
#14538=CARTESIAN_POINT ( 'NONE',  ( 43.29451156103230858, 3.885829148717482973, 6.335591667789099546 ) ) ;
#14539=CARTESIAN_POINT ( 'NONE',  ( 43.52775316163927499, 3.233996417830672154, 6.148606455994836573 ) ) ;
#14540=LINE ( 'NONE', #6813, #10259 ) ;
#14544=VERTEX_POINT ( 'NONE', #17512 ) ;
#14550=CARTESIAN_POINT ( 'NONE',  ( 32.81606138205700773, -35.82531359714782582, 71.25150419970752580 ) ) ;
#14582=ORIENTED_EDGE ( 'NONE', *, *, #3445, .F. ) ;
#14587=SHAPE_REPRESENTATION ( 'Follower', ( #2000 ), #17034 ) ;
#14594=CARTESIAN_POINT ( 'NONE',  ( 33.31606138205700773, -34.55876147765707174, 70.30501292736873609 ) ) ;
#14598=DIRECTION ( 'NONE',  ( 0.000000000000000000, -0.8212051873014203363, -0.5706330172266926848 ) ) ;
#14612=CARTESIAN_POINT ( 'NONE',  ( 42.85693730032902238, 2.786099971025956190, 6.091850983466585490 ) ) ;
#14634=DIRECTION ( 'NONE',  ( 0.000000000000000000, -0.4278636397681519488, 0.9038432971286277651 ) ) ;
#14639=ORIENTED_EDGE ( 'NONE', *, *, #22713, .T. ) ;
#14640=EDGE_LOOP ( 'NONE', ( #5843, #25314, #20428, #3867 ) ) ;
#14645=VERTEX_POINT ( 'NONE', #2663 ) ;
#14656=CARTESIAN_POINT ( 'NONE',  ( 43.20275628853117666, 3.610264363385236930, 6.334189765992617183 ) ) ;
#14657=CARTESIAN_POINT ( 'NONE',  ( 36.06606138205700063, 5.308699250829721272, 2.416607620847027960 ) ) ;
#14671=DIRECTION ( 'NONE',  ( 0.000000000000000000, -0.5706330172266952383, 0.8212051873014186709 ) ) ;
#14680=VECTOR ( 'NONE', #6246, 999.9999999999998863 ) ;
#14686=DIRECTION ( 'NONE',  ( 1.849283715844614949E-16, -0.8212051873014210024, -0.5706330172266920187 ) ) ;
#14709=CARTESIAN_POINT ( 'NONE',  ( 43.81606138205700063, 3.151453266960317023, 6.397347472316774031 ) ) ;
#14718=CARTESIAN_POINT ( 'NONE',  ( 32.81606138205700773, 2.740850673309605412, 6.112030963703427133 ) ) ;
#14719=PLANE ( 'NONE',  #23333 ) ;
#14732=ORIENTED_EDGE ( 'NONE', *, *, #17892, .T. ) ;
#14733=CARTESIAN_POINT ( 'NONE',  ( 40.06606138205700063, 6.004618353093779781, 2.291321535809666354 ) ) ;
#14741=CARTESIAN_POINT ( 'NONE',  ( 36.06606138205700063, 5.594015759443068170, 2.006005027196319901 ) ) ;
#14742=ORIENTED_EDGE ( 'NONE', *, *, #198, .F. ) ;
#14759=DIRECTION ( 'NONE',  ( 0.000000000000000000, 0.8212051873014210024, 0.5706330172266920187 ) ) ;
#14779=VECTOR ( 'NONE', #13943, 1000.000000000000000 ) ;
#14783=AXIS2_PLACEMENT_3D ( 'NONE', #6024, #9767, #4094 ) ;
#14818=AXIS2_PLACEMENT_3D ( 'NONE', #18416, #16464, #20217 ) ;
#14836=FACE_OUTER_BOUND ( 'NONE', #17024, .T. ) ;
#14852=CIRCLE ( 'NONE', #6642, 0.5000000000000004441 ) ;
#14856=VERTEX_POINT ( 'NONE', #3175 ) ;
#14865=CARTESIAN_POINT ( 'NONE',  ( 43.69896204258590444, 3.548173818309682037, 6.215045287937394747 ) ) ;
#14867=CARTESIAN_POINT ( 'NONE',  ( 33.31606138205700773, 0.9984178969752143251, 11.59873562314662010 ) ) ;
#14879=PLANE ( 'NONE',  #6688 ) ;
#14880=ORIENTED_EDGE ( 'NONE', *, *, #1124, .F. ) ;
#14906=FACE_OUTER_BOUND ( 'NONE', #13075, .T. ) ;
#14908=FACE_OUTER_BOUND ( 'NONE', #24118, .T. ) ;
#14909=CARTESIAN_POINT ( 'NONE',  ( 33.63430007298546087, 2.841684771932709186, 6.101742786271089791 ) ) ;
#14915=CARTESIAN_POINT ( 'NONE',  ( 32.81606138205700773, 6.705285648480822758, 7.416521610403067122 ) ) ;
#14934=CARTESIAN_POINT ( 'NONE',  ( 32.81606138205700773, -20.88462213363798270, 44.49284693533410717 ) ) ;
#14939=EDGE_CURVE ( 'NONE', #8708, #21114, #21465, .T. ) ;
#14945=VECTOR ( 'NONE', #2136, 1000.000000000000114 ) ;
#14947=LINE ( 'NONE', #15069, #25022 ) ;
#14949=AXIS2_PLACEMENT_3D ( 'NONE', #11262, #17053, #18980 ) ;
#14967=ORIENTED_EDGE ( 'NONE', *, *, #10564, .F. ) ;
#14981=DIRECTION ( 'NONE',  ( 1.000000000000000000, -0.000000000000000000, 0.000000000000000000 ) ) ;
#14982=FACE_OUTER_BOUND ( 'NONE', #8033, .T. ) ;
#14984=DIRECTION ( 'NONE',  ( 1.000000000000000000, -0.000000000000000000, 0.000000000000000000 ) ) ;
#14998=EDGE_LOOP ( 'NONE', ( #15690, #18751, #8672, #25145 ) ) ;
#15006=DIRECTION ( 'NONE',  ( 0.000000000000000000, -0.8212051873014210024, -0.5706330172266920187 ) ) ;
#15011=ADVANCED_FACE ( 'NONE', ( #25176 ), #39, .T. ) ;
#15016=ORIENTED_EDGE ( 'NONE', *, *, #1316, .T. ) ;
#15020=CARTESIAN_POINT ( 'NONE',  ( 34.06606138205700773, -32.75315594507191008, 59.38245422252773409 ) ) ;
#15027=LINE ( 'NONE', #1101, #16431 ) ;
#15039=CARTESIAN_POINT ( 'NONE',  ( 33.31606138205700773, -2.373793412309109563, 19.60611914621674146 ) ) ;
#15069=CARTESIAN_POINT ( 'NONE',  ( 33.40372220903689282, 3.256620197766214808, 6.241553153455755343 ) ) ;
#15073=ORIENTED_EDGE ( 'NONE', *, *, #20775, .T. ) ;
#15075=EDGE_CURVE ( 'NONE', #19555, #4227, #10640, .T. ) ;
#15077=EDGE_CURVE ( 'NONE', #22818, #19683, #6392, .T. ) ;
#15104=CARTESIAN_POINT ( 'NONE',  ( 33.09672011123848279, 3.247905043202620856, 6.142517800649935467 ) ) ;
#15107=VECTOR ( 'NONE', #17112, 1000.000000000000000 ) ;
#15117=DIRECTION ( 'NONE',  ( -1.000000000000000000, 0.000000000000000000, 0.000000000000000000 ) ) ;
#15123=CARTESIAN_POINT ( 'NONE',  ( 33.31606138205700773, -20.88462213363798270, 44.49284693533410717 ) ) ;
#15129=AXIS2_PLACEMENT_3D ( 'NONE', #17499, #15166, #1750 ) ;
#15137=SURFACE_STYLE_FILL_AREA ( #11544 ) ;
#15161=CARTESIAN_POINT ( 'NONE',  ( 42.99362139871320210, 2.839053109165292632, 6.102835131782519795 ) ) ;
#15166=DIRECTION ( 'NONE',  ( 1.425933913527082566E-16, -0.9038432971286278761, -0.4278636397681519488 ) ) ;
#15170=DIRECTION ( 'NONE',  ( 0.000000000000000000, -0.5706330172266913525, 0.8212051873014213355 ) ) ;
#15175=ORIENTED_EDGE ( 'NONE', *, *, #3655, .F. ) ;
#15197=ORIENTED_EDGE ( 'NONE', *, *, #4054, .T. ) ;
#15201=ORIENTED_EDGE ( 'NONE', *, *, #14232, .F. ) ;
#15209=VECTOR ( 'NONE', #13932, 1000.000000000000000 ) ;
#15225=AXIS2_PLACEMENT_3D ( 'NONE', #7934, #23877, #300 ) ;
#15231=CARTESIAN_POINT ( 'NONE',  ( 32.85323118609060344, 3.754743573466622575, 6.231177976620378978 ) ) ;
#15234=DIRECTION ( 'NONE',  ( 0.000000000000000000, 0.5706330172266915746, -0.8212051873014213355 ) ) ;
#15235=B_SPLINE_CURVE_WITH_KNOTS ( 'NONE', 3,
 ( #14338, #22193, #4795, #14223 ),
 .UNSPECIFIED., .F., .F.,
 ( 4, 4 ),
 ( 0.000000000000000000, 1.000000000000000000 ),
 .UNSPECIFIED. ) ;
#15257=CARTESIAN_POINT ( 'NONE',  ( 43.47464771180118248, 3.634064700962194028, 6.274728512395983948 ) ) ;
#15258=EDGE_CURVE ( 'NONE', #4551, #11492, #12955, .T. ) ;
#15266=CYLINDRICAL_SURFACE ( 'NONE', #4637, 0.4999999999999982792 ) ;
#15278=CARTESIAN_POINT ( 'NONE',  ( 33.31606138205700773, 4.124002793203064066, 6.312068993173404863 ) ) ;
#15281=ORIENTED_EDGE ( 'NONE', *, *, #18856, .F. ) ;
#15287=AXIS2_PLACEMENT_3D ( 'NONE', #8651, #6453, #12015 ) ;
#15297=ADVANCED_FACE ( 'NONE', ( #24892 ), #11146, .F. ) ;
#15302=CARTESIAN_POINT ( 'NONE',  ( 43.81606138205700063, -27.66931681479738003, 59.51410614687260647 ) ) ;
#15309=CARTESIAN_POINT ( 'NONE',  ( 42.82259846190797248, 3.224889648804766473, 6.370942050318627814 ) ) ;
#15317=VECTOR ( 'NONE', #6430, 1000.000000000000000 ) ;
#15328=ORIENTED_EDGE ( 'NONE', *, *, #12367, .F. ) ;
#15333=ORIENTED_EDGE ( 'NONE', *, *, #3578, .F. ) ;
#15345=CARTESIAN_POINT ( 'NONE',  ( 43.81606138205700063, -33.70281195181703993, 69.07320514641659770 ) ) ;
#15358=CARTESIAN_POINT ( 'NONE',  ( 33.56815104093937663, 3.421967759159691536, 6.351335392992072393 ) ) ;
#15389=EDGE_CURVE ( 'NONE', #8119, #24709, #13293, .T. ) ;
#15390=PLANE ( 'NONE',  #16313 ) ;
#15392=ADVANCED_FACE ( 'NONE', ( #18743 ), #3530, .T. ) ;
#15395=FILL_AREA_STYLE_COLOUR ( '', #11293 ) ;
#15425=LINE ( 'NONE', #23274, #7303 ) ;
#15426=CYLINDRICAL_SURFACE ( 'NONE', #22730, 0.7500000000000031086 ) ;
#15435=ORIENTED_EDGE ( 'NONE', *, *, #17196, .T. ) ;
#15446=ORIENTED_EDGE ( 'NONE', *, *, #2322, .F. ) ;
#15448=CARTESIAN_POINT ( 'NONE',  ( 33.31606138205700773, -4.962695059250739504, 17.19830099227260689 ) ) ;
#15457=CARTESIAN_POINT ( 'NONE',  ( 33.31606138205700773, -20.26871824316192061, 44.92082169825412308 ) ) ;
#15458=ORIENTED_EDGE ( 'NONE', *, *, #20566, .T. ) ;
#15483=CARTESIAN_POINT ( 'NONE',  ( 33.31606138205700773, 4.124002793203064066, 6.312068993173404863 ) ) ;
#15485=CARTESIAN_POINT ( 'NONE',  ( 40.06606138205700063, 5.308699250829721272, 2.416607620847027960 ) ) ;
#15489=ORIENTED_EDGE ( 'NONE', *, *, #15075, .F. ) ;
#15493=CARTESIAN_POINT ( 'NONE',  ( 33.31606138205700773, 6.366250835946940967, 6.636353555660927661 ) ) ;
#15542=CARTESIAN_POINT ( 'NONE',  ( 43.39072112804083758, 3.102161780315297435, 6.136388117020254107 ) ) ;
#15555=ORIENTED_EDGE ( 'NONE', *, *, #15832, .F. ) ;
#15560=EDGE_CURVE ( 'NONE', #22410, #10213, #5718, .T. ) ;
#15569=DIRECTION ( 'NONE',  ( 1.000000000000000000, -0.000000000000000000, 0.000000000000000000 ) ) ;
#15602=DIRECTION ( 'NONE',  ( 1.000000000000000000, 0.000000000000000000, 0.000000000000000000 ) ) ;
#15605=EDGE_LOOP ( 'NONE', ( #16495, #9782, #1603, #24137 ) ) ;
#15606=CARTESIAN_POINT ( 'NONE',  ( 43.81606138205700063, -27.66931681479738003, 59.51410614687260647 ) ) ;
#15609=CARTESIAN_POINT ( 'NONE',  ( 33.34326309846886005, 3.870673299598025086, 6.311734371576938507 ) ) ;
#15617=CARTESIAN_POINT ( 'NONE',  ( 38.31606138205700063, -6.549308025893449070, 20.35783565644092619 ) ) ;
#15634=CARTESIAN_POINT ( 'NONE',  ( 43.31606138205700063, -27.52349462642295208, 56.67559192035834315 ) ) ;
#15639=VECTOR ( 'NONE', #21787, 1000.000000000000000 ) ;
#15640=FACE_OUTER_BOUND ( 'NONE', #11794, .T. ) ;
#15641=ORIENTED_EDGE ( 'NONE', *, *, #17759, .T. ) ;
#15664=DIRECTION ( 'NONE',  ( 1.000000000000000000, 1.159780179694326360E-16, 8.617271610285116919E-17 ) ) ;
#15669=CARTESIAN_POINT ( 'NONE',  ( 42.82259739205072435, 3.224889171211050343, 6.370942055173422602 ) ) ;
#15678=LINE ( 'NONE', #2267, #16758 ) ;
#15679=CARTESIAN_POINT ( 'NONE',  ( 43.31606138205700063, -20.88462213363798270, 44.49284693533410717 ) ) ;
#15682=B_SPLINE_SURFACE_WITH_KNOTS ( 'NONE', 1, 3, ( 
 ( #18286, #12229, #23802, #4366 ),
 ( #2166, #19953, #14277, #8615 ),
 ( #21885, #18402, #350, #14163 ) ),
 .UNSPECIFIED., .F., .F., .F.,
 ( 2, 1, 2 ),
 ( 4, 4 ),
 ( -0.01000000000000000021, 0.000000000000000000, 1.000000000000000000 ),
 ( 0.000000000000000000, 1.000000000000000000 ),
 .UNSPECIFIED. ) ;
#15684=ORIENTED_EDGE ( 'NONE', *, *, #3412, .T. ) ;
#15690=ORIENTED_EDGE ( 'NONE', *, *, #20148, .T. ) ;
#15704=ADVANCED_FACE ( 'NONE', ( #23984 ), #538, .F. ) ;
#15708=CYLINDRICAL_SURFACE ( 'NONE', #24407, 0.5000000000000011102 ) ;
#15713=ORIENTED_EDGE ( 'NONE', *, *, #15560, .T. ) ;
#15728=APPLICATION_CONTEXT ( 'automotive_design' ) ;
#15748=CARTESIAN_POINT ( 'NONE',  ( 38.31606138205700063, 5.594015759443068170, 2.006005027196319901 ) ) ;
#15751=ORIENTED_EDGE ( 'NONE', *, *, #22713, .F. ) ;
#15764=VECTOR ( 'NONE', #3758, 1000.000000000000114 ) ;
#15766=FACE_OUTER_BOUND ( 'NONE', #8127, .T. ) ;
#15769=DIRECTION ( 'NONE',  ( 0.000000000000000000, -0.5706330172266920187, 0.8212051873014210024 ) ) ;
#15795=CARTESIAN_POINT ( 'NONE',  ( 33.32114655809477455, -33.12114953149414021, 59.73560708446382250 ) ) ;
#15805=ORIENTED_EDGE ( 'NONE', *, *, #7148, .T. ) ;
#15806=CARTESIAN_POINT ( 'NONE',  ( 43.31606138205700063, 4.103895195095678794, 6.341006091748962348 ) ) ;
#15813=DIRECTION ( 'NONE',  ( -1.000000000000000000, 0.000000000000000000, 0.000000000000000000 ) ) ;
#15816=B_SPLINE_CURVE_WITH_KNOTS ( 'NONE', 3,
 ( #6811, #24555, #6936, #20725 ),
 .UNSPECIFIED., .F., .F.,
 ( 4, 4 ),
 ( 0.000000000000000000, 1.000000000000000000 ),
 .UNSPECIFIED. ) ;
#15817=CARTESIAN_POINT ( 'NONE',  ( 43.39709375099405975, 3.108381023609500193, 6.137326095127844994 ) ) ;
#15828=CARTESIAN_POINT ( 'NONE',  ( 34.06606138205700773, -37.53049398575952722, 70.06662099985003067 ) ) ;
#15832=EDGE_CURVE ( 'NONE', #20815, #5208, #6851, .T. ) ;
#15836=ORIENTED_EDGE ( 'NONE', *, *, #5648, .T. ) ;
#15838=DIRECTION ( 'NONE',  ( 0.000000000000000000, -0.5706330172266952383, 0.8212051873014186709 ) ) ;
#15852=DIRECTION ( 'NONE',  ( 0.000000000000000000, 0.5706330172266907974, -0.8212051873014217795 ) ) ;
#15856=EDGE_CURVE ( 'NONE', #24417, #25393, #10861, .T. ) ;
#15870=DIRECTION ( 'NONE',  ( -1.734723475976804876E-16, 0.8212051873014210024, 0.5706330172266920187 ) ) ;
#15886=PRODUCT_DEFINITION_SHAPE ( 'NONE', 'NONE',  #2830 ) ;
#15896=EDGE_LOOP ( 'NONE', ( #6957, #24995, #6814, #8035 ) ) ;
#15902=ORIENTED_EDGE ( 'NONE', *, *, #7602, .F. ) ;
#15906=ORIENTED_EDGE ( 'NONE', *, *, #22249, .F. ) ;
#15915=LINE ( 'NONE', #12074, #9945 ) ;
#15926=DIRECTION ( 'NONE',  ( -1.000000000000000000, 0.000000000000000000, 0.000000000000000000 ) ) ;
#15933=EDGE_CURVE ( 'NONE', #20004, #23532, #3847, .T. ) ;
#15950=VECTOR ( 'NONE', #18063, 1000.000000000000114 ) ;
#15951=CARTESIAN_POINT ( 'NONE',  ( 32.81606138205700063, 3.939336499464421770, 6.271597994279004773 ) ) ;
#15959=CARTESIAN_POINT ( 'NONE',  ( 32.81606138205700773, -37.34243788671330577, 70.80615726751818784 ) ) ;
#15964=VECTOR ( 'NONE', #23147, 1000.000000000000114 ) ;
#15968=LINE ( 'NONE', #2562, #19244 ) ;
#15990=CIRCLE ( 'NONE', #3653, 0.7500000000000031086 ) ;
#16024=EDGE_CURVE ( 'NONE', #1658, #2590, #13800, .T. ) ;
#16025=CARTESIAN_POINT ( 'NONE',  ( 33.31606138205700773, -33.60910547091194900, 60.61426200347987248 ) ) ;
#16041=CARTESIAN_POINT ( 'NONE',  ( 43.81606138205700063, -37.34243788671330577, 70.80615726751818784 ) ) ;
#16046=VECTOR ( 'NONE', #8017, 1000.000000000000114 ) ;
#16052=CARTESIAN_POINT ( 'NONE',  ( 43.31606138205700063, -20.88462213363798270, 44.49284693533410717 ) ) ;
#16056=CARTESIAN_POINT ( 'NONE',  ( 32.81606138205700773, -33.60910547091194900, 60.61426200347987248 ) ) ;
#16060=FACE_OUTER_BOUND ( 'NONE', #5369, .T. ) ;
#16061=CARTESIAN_POINT ( 'NONE',  ( 43.31606138205700063, -21.31259689655800216, 45.10875082581016926 ) ) ;
#16098=ORIENTED_EDGE ( 'NONE', *, *, #22406, .T. ) ;
#16100=DIRECTION ( 'NONE',  ( 1.000000000000000000, 0.000000000000000000, 0.000000000000000000 ) ) ;
#16105=EDGE_CURVE ( 'NONE', #22104, #5709, #9625, .T. ) ;
#16112=DIRECTION ( 'NONE',  ( -1.000000000000000000, -1.187136597504755470E-16, -8.249087426255173666E-17 ) ) ;
#16116=EDGE_CURVE ( 'NONE', #13605, #22410, #10844, .T. ) ;
#16137=VECTOR ( 'NONE', #18782, 1000.000000000000114 ) ;
#16139=CARTESIAN_POINT ( 'NONE',  ( 43.81606138205700063, -27.11289203277224402, 56.96090842897168471 ) ) ;
#16156=AXIS2_PLACEMENT_3D ( 'NONE', #14509, #14759, #12717 ) ;
#16157=LINE ( 'NONE', #24009, #922 ) ;
#16162=VERTEX_POINT ( 'NONE', #2064 ) ;
#16166=LINE ( 'NONE', #6394, #24307 ) ;
#16172=AXIS2_PLACEMENT_3D ( 'NONE', #16851, #4745, #12863 ) ;
#16184=LINE ( 'NONE', #14383, #5446 ) ;
#16218=COLOUR_RGB ( '', 0.72549020, 0.75294118, 0.79215686) ;
#16224=ADVANCED_FACE ( 'NONE', ( #4271 ), #374, .F. ) ;
#16226=ADVANCED_FACE ( 'NONE', ( #4395 ), #23705, .T. ) ;
#16233=CARTESIAN_POINT ( 'NONE',  ( 43.31606138205700063, -38.37466412126273951, 70.68129701848354784 ) ) ;
#16234=CARTESIAN_POINT ( 'NONE',  ( 42.99361969242278292, 2.839052459004266726, 6.102834979010582472 ) ) ;
#16254=EDGE_LOOP ( 'NONE', ( #4825, #14742, #7455, #18262 ) ) ;
#16259=VERTEX_POINT ( 'NONE', #16234 ) ;
#16266=LINE ( 'NONE', #10229, #3606 ) ;
#16273=CARTESIAN_POINT ( 'NONE',  ( 34.06606138205700773, 2.740850673309605412, 6.112030963703427133 ) ) ;
#16277=EDGE_LOOP ( 'NONE', ( #11182, #21194, #2740, #3943 ) ) ;
#16286=ORIENTED_EDGE ( 'NONE', *, *, #15832, .T. ) ;
#16287=CARTESIAN_POINT ( 'NONE',  ( 32.81606138205700773, -33.60910547091194900, 60.61426200347987248 ) ) ;
#16290=DIRECTION ( 'NONE',  ( 0.000000000000000000, -0.8212051873014203363, -0.5706330172266926848 ) ) ;
#16304=EDGE_CURVE ( 'NONE', #12100, #25424, #22769, .T. ) ;
#16309=ORIENTED_EDGE ( 'NONE', *, *, #12407, .T. ) ;
#16313=AXIS2_PLACEMENT_3D ( 'NONE', #11922, #19380, #17463 ) ;
#16326=CIRCLE ( 'NONE', #21670, 0.5000000000000004441 ) ;
#16329=VECTOR ( 'NONE', #16667, 1000.000000000000000 ) ;
#16331=DIRECTION ( 'NONE',  ( 0.000000000000000000, 0.5706330172266920187, -0.8212051873014210024 ) ) ;
#16349=CARTESIAN_POINT ( 'NONE',  ( 43.31606138205700063, 6.289375473607850431, 7.138843309009015314 ) ) ;
#16353=CARTESIAN_POINT ( 'NONE',  ( 33.23058527440272059, 3.113468987225112006, 6.136968036621317069 ) ) ;
#16363=AXIS2_PLACEMENT_3D ( 'NONE', #9851, #15769, #3410 ) ;
#16370=ORIENTED_EDGE ( 'NONE', *, *, #13126, .T. ) ;
#16398=CIRCLE ( 'NONE', #3661, 0.4999999999999982792 ) ;
#16414=ORIENTED_EDGE ( 'NONE', *, *, #23591, .F. ) ;
#16415=CARTESIAN_POINT ( 'NONE',  ( 33.31606138205700773, 3.996716213179724697, 6.311483552851885115 ) ) ;
#16431=VECTOR ( 'NONE', #13110, 1000.000000000000227 ) ;
#16456=VECTOR ( 'NONE', #633, 1000.000000000000114 ) ;
#16464=DIRECTION ( 'NONE',  ( 0.000000000000000000, -0.5706330172266920187, 0.8212051873014210024 ) ) ;
#16473=ORIENTED_EDGE ( 'NONE', *, *, #3655, .T. ) ;
#16490=CARTESIAN_POINT ( 'NONE',  ( 43.31606138205700063, 0.9984178969752143251, 11.59873562314662010 ) ) ;
#16495=ORIENTED_EDGE ( 'NONE', *, *, #23237, .F. ) ;
#16498=DIRECTION ( 'NONE',  ( 1.000000000000000000, -0.000000000000000000, 0.000000000000000000 ) ) ;
#16514=DIRECTION ( 'NONE',  ( -1.000000000000000000, 0.000000000000000000, 0.000000000000000000 ) ) ;
#16516=CYLINDRICAL_SURFACE ( 'NONE', #12941, 2.500000000000002220 ) ;
#16532=ORIENTED_EDGE ( 'NONE', *, *, #13756, .F. ) ;
#16543=DIRECTION ( 'NONE',  ( 1.000000000000000000, 0.000000000000000000, 0.000000000000000000 ) ) ;
#16547=DIRECTION ( 'NONE',  ( -1.000000000000000000, 0.000000000000000000, 0.000000000000000000 ) ) ;
#16550=ORIENTED_EDGE ( 'NONE', *, *, #4521, .T. ) ;
#16556=VECTOR ( 'NONE', #8996, 1000.000000000000114 ) ;
#16575=ORIENTED_EDGE ( 'NONE', *, *, #17907, .F. ) ;
#16587=AXIS2_PLACEMENT_3D ( 'NONE', #8259, #14431, #16100 ) ;
#16589=CYLINDRICAL_SURFACE ( 'NONE', #7919, 1.499999999999996669 ) ;
#16590=LINE ( 'NONE', #9007, #366 ) ;
#16593=PLANE ( 'NONE',  #2021 ) ;
#16595=DIRECTION ( 'NONE',  ( 0.000000000000000000, 0.5706330172266919076, -0.8212051873014208914 ) ) ;
#16606=VERTEX_POINT ( 'NONE', #5536 ) ;
#16608=CARTESIAN_POINT ( 'NONE',  ( 43.31606138205700063, -27.11289203277224402, 56.96090842897168471 ) ) ;
#16616=EDGE_CURVE ( 'NONE', #19555, #18958, #7721, .T. ) ;
#16626=CARTESIAN_POINT ( 'NONE',  ( 33.72038411900453525, 3.276404855341403355, 6.354292672466786307 ) ) ;
#16627=ORIENTED_EDGE ( 'NONE', *, *, #25130, .F. ) ;
#16630=DIRECTION ( 'NONE',  ( 0.000000000000000000, 0.8212051873014208914, 0.5706330172266919076 ) ) ;
#16645=FACE_BOUND ( 'NONE', #9427, .T. ) ;
#16653=EDGE_CURVE ( 'NONE', #7328, #2134, #967, .T. ) ;
#16656=ORIENTED_EDGE ( 'NONE', *, *, #109, .F. ) ;
#16667=DIRECTION ( 'NONE',  ( -1.000000000000000000, -1.187136597504755470E-16, -8.249087426255173666E-17 ) ) ;
#16680=DIRECTION ( 'NONE',  ( -1.000000000000000000, 1.508529456107831862E-16, 1.048235847051697233E-16 ) ) ;
#16682=DIRECTION ( 'NONE',  ( -2.168404344971010101E-16, 0.8212051873014210024, 0.5706330172266920187 ) ) ;
#16687=ORIENTED_EDGE ( 'NONE', *, *, #10244, .T. ) ;
#16729=ORIENTED_EDGE ( 'NONE', *, *, #2858, .F. ) ;
#16730=UNCERTAINTY_MEASURE_WITH_UNIT (LENGTH_MEASURE( 1.000000000000000082E-05 ), #11026, 'distance_accuracy_value', 'NONE');
#16737=ORIENTED_EDGE ( 'NONE', *, *, #13974, .F. ) ;
#16741=AXIS2_PLACEMENT_3D ( 'NONE', #4718, #17876, #10261 ) ;
#16742=VERTEX_POINT ( 'NONE', #14253 ) ;
#16743=CARTESIAN_POINT ( 'NONE',  ( 43.81606138205700063, -39.23120981750657421, 69.49370132789680099 ) ) ;
#16753=EDGE_LOOP ( 'NONE', ( #21607, #7975, #20834, #3218, #4776, #3143, #17563, #7666, #15197, #10530 ) ) ;
#16757=AXIS2_PLACEMENT_3D ( 'NONE', #22960, #20911, #20523 ) ;
#16758=VECTOR ( 'NONE', #17883, 1000.000000000000000 ) ;
#16763=ORIENTED_EDGE ( 'NONE', *, *, #13490, .F. ) ;
#16767=ORIENTED_EDGE ( 'NONE', *, *, #18309, .T. ) ;
#16794=VERTEX_POINT ( 'NONE', #22731 ) ;
#16810=DIRECTION ( 'NONE',  ( 0.000000000000000000, -0.5706330172266915746, 0.8212051873014213355 ) ) ;
#16819=ORIENTED_EDGE ( 'NONE', *, *, #11618, .T. ) ;
#16821=ADVANCED_FACE ( 'NONE', ( #18748 ), #5470, .F. ) ;
#16831=EDGE_CURVE ( 'NONE', #1002, #22555, #1080, .T. ) ;
#16849=CARTESIAN_POINT ( 'NONE',  ( 34.06606138205700773, -37.81581049437287589, 70.47722359350073873 ) ) ;
#16851=CARTESIAN_POINT ( 'NONE',  ( 33.31606138205700773, 6.294683054830111146, 7.131205101789720224 ) ) ;
#16853=DIRECTION ( 'NONE',  ( 1.000000000000000000, -3.299634970502069713E-17, 4.748546390019022251E-17 ) ) ;
#16855=CIRCLE ( 'NONE', #23426, 0.5000000000000004441 ) ;
#16869=EDGE_CURVE ( 'NONE', #14544, #13705, #13215, .T. ) ;
#16883=VECTOR ( 'NONE', #24598, 1000.000000000000114 ) ;
#16885=EDGE_CURVE ( 'NONE', #19940, #2302, #1212, .T. ) ;
#16892=ORIENTED_EDGE ( 'NONE', *, *, #10224, .T. ) ;
#16896=ORIENTED_EDGE ( 'NONE', *, *, #19347, .T. ) ;
#16900=ADVANCED_FACE ( 'NONE', ( #24643 ), #7021, .T. ) ;
#16907=MANIFOLD_SOLID_BREP ( 'NONE', #11017 ) ;
#16918=DIRECTION ( 'NONE',  ( -1.000000000000000000, -1.185941393278724777E-16, -8.240782279085522416E-17 ) ) ;
#16937=CARTESIAN_POINT ( 'NONE',  ( 43.31606138205700063, 3.973594872748516416, 6.337251443159059860 ) ) ;
#16941=DIRECTION ( 'NONE',  ( -1.000000000000000000, 0.000000000000000000, 0.000000000000000000 ) ) ;
#16953=CARTESIAN_POINT ( 'NONE',  ( 33.80700705136447937, 3.227014435054107455, 6.369498925975481285 ) ) ;
#16974=EDGE_CURVE ( 'NONE', #3435, #16742, #17062, .T. ) ;
#16975=ADVANCED_FACE ( 'NONE', ( #15766 ), #23624, .T. ) ;
#16981=CARTESIAN_POINT ( 'NONE',  ( 42.56606138205700063, -39.60075215179220720, 69.23691647014479145 ) ) ;
#17021=CARTESIAN_POINT ( 'NONE',  ( 43.81606138205700063, -35.70002751211045933, 71.94742330197156832 ) ) ;
#17023=VECTOR ( 'NONE', #10734, 1000.000000000000000 ) ;
#17024=EDGE_LOOP ( 'NONE', ( #2377, #7162, #11843, #19590, #15555, #4415, #13697, #3990, #16627, #24309 ) ) ;
#17034=( GEOMETRIC_REPRESENTATION_CONTEXT ( 3 ) GLOBAL_UNCERTAINTY_ASSIGNED_CONTEXT ( ( #16730 ) ) GLOBAL_UNIT_ASSIGNED_CONTEXT ( ( #11026, #22869, #8237 ) ) REPRESENTATION_CONTEXT ( 'NONE', 'WORKASPACE' ) );
#17037=FACE_BOUND ( 'NONE', #13015, .T. ) ;
#17053=DIRECTION ( 'NONE',  ( 0.000000000000000000, 0.5706330172266920187, -0.8212051873014210024 ) ) ;
#17062=CIRCLE ( 'NONE', #9663, 0.7500000000000031086 ) ;
#17073=ADVANCED_FACE ( 'NONE', ( #6231 ), #12172, .T. ) ;
#17087=CARTESIAN_POINT ( 'NONE',  ( 43.31606138205700063, -27.60498114914042134, 57.04949906928994352 ) ) ;
#17088=VERTEX_POINT ( 'NONE', #792 ) ;
#17097=AXIS2_PLACEMENT_3D ( 'NONE', #14934, #3203, #22665 ) ;
#17098=LINE ( 'NONE', #20704, #23534 ) ;
#17099=LINE ( 'NONE', #10918, #25486 ) ;
#17112=DIRECTION ( 'NONE',  ( 1.000000000000000000, -0.000000000000000000, 0.000000000000000000 ) ) ;
#17113=LINE ( 'NONE', #3057, #16137 ) ;
#17118=B_SPLINE_SURFACE_WITH_KNOTS ( 'NONE', 1, 3, ( 
 ( #21285, #9331, #7765, #17175, #15104, #13061 ),
 ( #5326, #25124, #15231, #3628, #17428, #7641 ),
 ( #15483, #23331, #13188, #25383, #5697, #13561 ),
 ( #17304, #13316, #15609, #7506, #11640, #15358 ) ),
 .UNSPECIFIED., .F., .F., .F.,
 ( 2, 1, 1, 2 ),
 ( 4, 2, 4 ),
 ( -0.01000000000000000021, 0.000000000000000000, 1.000000000000000000, 1.010099999999999998 ),
 ( 0.000000000000000000, 0.5000000000000000000, 1.000000000000000000 ),
 .UNSPECIFIED. ) ;
#17127=EDGE_CURVE ( 'NONE', #2353, #18040, #20140, .T. ) ;
#17138=EDGE_CURVE ( 'NONE', #12100, #17728, #14088, .T. ) ;
#17170=CARTESIAN_POINT ( 'NONE',  ( 43.31606138205700063, 3.172506336381830661, 12.50058896911730066 ) ) ;
#17172=LINE ( 'NONE', #13556, #22518 ) ;
#17175=CARTESIAN_POINT ( 'NONE',  ( 32.99125882899717510, 3.408086086664901870, 6.165992285920837368 ) ) ;
#17179=DIRECTION ( 'NONE',  ( 1.000000000000000000, -0.000000000000000000, 0.000000000000000000 ) ) ;
#17192=CARTESIAN_POINT ( 'NONE',  ( 43.82106138205700319, 4.103895195095678794, 6.341006091748962348 ) ) ;
#17196=EDGE_CURVE ( 'NONE', #24226, #18636, #15235, .T. ) ;
#17209=ORIENTED_EDGE ( 'NONE', *, *, #15933, .T. ) ;
#17225=VERTEX_POINT ( 'NONE', #7377 ) ;
#17231=CARTESIAN_POINT ( 'NONE',  ( 42.74055771317608787, 3.188265934946779012, 6.371314334530746137 ) ) ;
#17238=ADVANCED_FACE ( 'NONE', ( #12674 ), #2849, .F. ) ;
#17248=AXIS2_PLACEMENT_3D ( 'NONE', #20242, #12536, #12402 ) ;
#17256=VERTEX_POINT ( 'NONE', #3238 ) ;
#17261=AXIS2_PLACEMENT_3D ( 'NONE', #15302, #22781, #20852 ) ;
#17271=LINE ( 'NONE', #9930, #6171 ) ;
#17284=ADVANCED_FACE ( 'NONE', ( #5315 ), #22698, .T. ) ;
#17291=EDGE_CURVE ( 'NONE', #22414, #24159, #7902, .T. ) ;
#17304=CARTESIAN_POINT ( 'NONE',  ( 33.32111138205700485, 4.124002793203064066, 6.312068993173404863 ) ) ;
#17311=ORIENTED_EDGE ( 'NONE', *, *, #6981, .F. ) ;
#17313=ORIENTED_EDGE ( 'NONE', *, *, #18156, .T. ) ;
#17314=LINE ( 'NONE', #13445, #9468 ) ;
#17316=CIRCLE ( 'NONE', #5380, 0.5000000000000000000 ) ;
#17324=( NAMED_UNIT ( * ) PLANE_ANGLE_UNIT ( ) SI_UNIT ( $, .RADIAN. ) );
#17325=B_SPLINE_SURFACE_WITH_KNOTS ( 'NONE', 1, 3, ( 
 ( #18991, #1332, #3135, #5083 ),
 ( #8951, #25010, #7141, #9218 ) ),
 .UNSPECIFIED., .F., .F., .F.,
 ( 2, 2 ),
 ( 4, 4 ),
 ( 0.000000000000000000, 1.000000000000000000 ),
 ( 0.000000000000000000, 1.000000000000000000 ),
 .UNSPECIFIED. ) ;
#17326=PLANE ( 'NONE',  #16363 ) ;
#17328=LINE ( 'NONE', #1348, #3017 ) ;
#17335=EDGE_LOOP ( 'NONE', ( #6625, #8289, #14880, #4037 ) ) ;
#17344=ORIENTED_EDGE ( 'NONE', *, *, #422, .T. ) ;
#17351=ORIENTED_EDGE ( 'NONE', *, *, #20305, .F. ) ;
#17371=CARTESIAN_POINT ( 'NONE',  ( 43.81606138205700063, -36.11063010576116739, 71.66210679335823386 ) ) ;
#17428=CARTESIAN_POINT ( 'NONE',  ( 33.10058206061923869, 3.250575416431807696, 6.144373406101647284 ) ) ;
#17436=ADVANCED_FACE ( 'NONE', ( #18056 ), #10077, .T. ) ;
#17453=EDGE_CURVE ( 'NONE', #9754, #18371, #11884, .T. ) ;
#17454=LINE ( 'NONE', #19242, #10236 ) ;
#17460=EDGE_LOOP ( 'NONE', ( #8186, #7057, #20350, #19542 ) ) ;
#17461=LINE ( 'NONE', #9358, #11265 ) ;
#17463=DIRECTION ( 'NONE',  ( 1.000000000000000000, -0.000000000000000000, 0.000000000000000000 ) ) ;
#17489=EDGE_CURVE ( 'NONE', #21396, #24541, #5414, .T. ) ;
#17499=CARTESIAN_POINT ( 'NONE',  ( 32.81606138205700773, -32.95845724189726411, 59.23979596822106686 ) ) ;
#17503=AXIS2_PLACEMENT_3D ( 'NONE', #16233, #6449, #18427 ) ;
#17512=CARTESIAN_POINT ( 'NONE',  ( 43.31606138205700063, -36.11063010576116739, 71.66210679335823386 ) ) ;
#17563=ORIENTED_EDGE ( 'NONE', *, *, #7692, .F. ) ;
#17577=( NAMED_UNIT ( * ) SI_UNIT ( $, .STERADIAN. ) SOLID_ANGLE_UNIT ( ) );
#17591=EDGE_CURVE ( 'NONE', #170, #1658, #12773, .T. ) ;
#17597=VERTEX_POINT ( 'NONE', #8777 ) ;
#17606=DIRECTION ( 'NONE',  ( 1.849283715844614702E-16, -0.8212051873014210024, -0.5706330172266920187 ) ) ;
#17627=CARTESIAN_POINT ( 'NONE',  ( 43.81608638205700146, -2.373793412309109563, 19.60611914621674146 ) ) ;
#17645=ORIENTED_EDGE ( 'NONE', *, *, #9738, .F. ) ;
#17657=DIRECTION ( 'NONE',  ( 0.000000000000000000, 0.5706330172266919076, -0.8212051873014208914 ) ) ;
#17669=PLANE ( 'NONE',  #10588 ) ;
#17714=CARTESIAN_POINT ( 'NONE',  ( 33.35568666798391746, 2.997371002701979759, 6.110935844446934162 ) ) ;
#17728=VERTEX_POINT ( 'NONE', #12101 ) ;
#17740=ADVANCED_FACE ( 'NONE', ( #21875 ), #19943, .F. ) ;
#17743=EDGE_LOOP ( 'NONE', ( #1169, #10897, #14582, #6098 ) ) ;
#17745=VERTEX_POINT ( 'NONE', #340 ) ;
#17749=CARTESIAN_POINT ( 'NONE',  ( 43.81606138205700063, -33.60910547091194900, 60.61426200347987248 ) ) ;
#17759=EDGE_CURVE ( 'NONE', #25244, #9104, #4358, .T. ) ;
#17763=EDGE_CURVE ( 'NONE', #952, #22308, #24160, .T. ) ;
#17775=CYLINDRICAL_SURFACE ( 'NONE', #7766, 0.7500000000000031086 ) ;
#17778=DIRECTION ( 'NONE',  ( 0.000000000000000000, -0.5706330172266952383, 0.8212051873014186709 ) ) ;
#17795=ORIENTED_EDGE ( 'NONE', *, *, #4465, .T. ) ;
#17812=DIRECTION ( 'NONE',  ( 0.000000000000000000, -0.8212051873014186709, -0.5706330172266952383 ) ) ;
#17826=EDGE_LOOP ( 'NONE', ( #17645, #681, #1182, #12288 ) ) ;
#17853=CARTESIAN_POINT ( 'NONE',  ( 43.31606138205700063, -2.373793412309109563, 19.60611914621674146 ) ) ;
#17862=VERTEX_POINT ( 'NONE', #7041 ) ;
#17876=DIRECTION ( 'NONE',  ( 1.000000000000000000, -0.000000000000000000, 0.000000000000000000 ) ) ;
#17878=VECTOR ( 'NONE', #19794, 1000.000000000000000 ) ;
#17883=DIRECTION ( 'NONE',  ( 1.000000000000000000, -0.000000000000000000, 0.000000000000000000 ) ) ;
#17892=EDGE_CURVE ( 'NONE', #22308, #17597, #12462, .T. ) ;
#17907=EDGE_CURVE ( 'NONE', #17225, #4853, #17098, .T. ) ;
#17909=CARTESIAN_POINT ( 'NONE',  ( 36.06606138205700063, 6.004618353093779781, 2.291321535809666354 ) ) ;
#17913=DIRECTION ( 'NONE',  ( 0.000000000000000000, -0.8212051873014203363, -0.5706330172266926848 ) ) ;
#17915=DIRECTION ( 'NONE',  ( -1.000000000000000000, 0.000000000000000000, 0.000000000000000000 ) ) ;
#17922=ORIENTED_EDGE ( 'NONE', *, *, #199, .T. ) ;
#17948=EDGE_CURVE ( 'NONE', #6765, #22555, #12508, .T. ) ;
#17962=DIRECTION ( 'NONE',  ( -6.464932690748116116E-17, -0.1431355622335914179, 0.9897030922575081879 ) ) ;
#17968=EDGE_LOOP ( 'NONE', ( #16763, #11870, #3547, #13855 ) ) ;
#17990=ORIENTED_EDGE ( 'NONE', *, *, #3960, .T. ) ;
#18005=EDGE_CURVE ( 'NONE', #10314, #2590, #12253, .T. ) ;
#18006=CARTESIAN_POINT ( 'NONE',  ( 43.81606138205700063, -0.03546393544221274063, 20.62209909563275900 ) ) ;
#18033=EDGE_CURVE ( 'NONE', #25120, #13976, #13734, .T. ) ;
#18038=FACE_BOUND ( 'NONE', #468, .T. ) ;
#18040=VERTEX_POINT ( 'NONE', #15278 ) ;
#18043=ORIENTED_EDGE ( 'NONE', *, *, #9517, .F. ) ;
#18049=DIRECTION ( 'NONE',  ( -1.000000000000000000, 0.000000000000000000, 0.000000000000000000 ) ) ;
#18055=PLANE ( 'NONE',  #1643 ) ;
#18056=FACE_OUTER_BOUND ( 'NONE', #23637, .T. ) ;
#18063=DIRECTION ( 'NONE',  ( 0.000000000000000000, -0.8212051873014208914, -0.5706330172266919076 ) ) ;
#18073=DIRECTION ( 'NONE',  ( -1.000000000000000000, 0.000000000000000000, 0.000000000000000000 ) ) ;
#18076=ORIENTED_EDGE ( 'NONE', *, *, #11208, .T. ) ;
#18098=CARTESIAN_POINT ( 'NONE',  ( 33.48992690894276336, 2.908530785145326814, 6.098665089938691608 ) ) ;
#18103=EDGE_LOOP ( 'NONE', ( #16370, #23579, #12824, #8648 ) ) ;
#18116=CIRCLE ( 'NONE', #7423, 0.5000000000000011102 ) ;
#18123=CARTESIAN_POINT ( 'NONE',  ( 40.81606138205700773, -29.37462871496113337, 53.20604314849776983 ) ) ;
#18156=EDGE_CURVE ( 'NONE', #12466, #10938, #713, .T. ) ;
#18157=CARTESIAN_POINT ( 'NONE',  ( 43.27366112336382287, 3.802330592292169964, 6.334870612574754034 ) ) ;
#18168=LINE ( 'NONE', #15959, #2894 ) ;
#18180=CARTESIAN_POINT ( 'NONE',  ( 32.81606138205700773, -34.55876147765707174, 70.30501292736873609 ) ) ;
#18189=CARTESIAN_POINT ( 'NONE',  ( 43.24580177837434292, 3.721690752961227755, 6.335617458560805382 ) ) ;
#18192=CARTESIAN_POINT ( 'NONE',  ( 33.63983381732847988, 3.338985100189466149, 6.348312178689456964 ) ) ;
#18196=FACE_OUTER_BOUND ( 'NONE', #19233, .T. ) ;
#18228=CYLINDRICAL_SURFACE ( 'NONE', #4934, 0.7499999999999983347 ) ;
#18235=ORIENTED_EDGE ( 'NONE', *, *, #5767, .F. ) ;
#18245=CARTESIAN_POINT ( 'NONE',  ( 43.81606138205700063, -1.963190818658398173, 19.89143565483009013 ) ) ;
#18248=CARTESIAN_POINT ( 'NONE',  ( 33.31606138205700773, -35.82531359714782582, 71.25150419970752580 ) ) ;
#18262=ORIENTED_EDGE ( 'NONE', *, *, #25301, .F. ) ;
#18264=CARTESIAN_POINT ( 'NONE',  ( 43.31606138205700063, -35.70002751211045933, 71.94742330197156832 ) ) ;
#18265=VECTOR ( 'NONE', #19339, 1000.000000000000114 ) ;
#18267=DIRECTION ( 'NONE',  ( -1.000000000000000000, 0.000000000000000000, 0.000000000000000000 ) ) ;
#18268=CIRCLE ( 'NONE', #13320, 1.499999999999996669 ) ;
#18282=DIRECTION ( 'NONE',  ( 0.000000000000000000, -0.5706330172266919076, 0.8212051873014208914 ) ) ;
#18286=CARTESIAN_POINT ( 'NONE',  ( 42.99533221766311897, 2.835194994361335485, 6.100154078057893337 ) ) ;
#18293=CARTESIAN_POINT ( 'NONE',  ( 42.56606138205700063, -39.60075215179220720, 69.23691647014479145 ) ) ;
#18309=EDGE_CURVE ( 'NONE', #7627, #11457, #11270, .T. ) ;
#18312=DIRECTION ( 'NONE',  ( 0.000000000000000000, 0.5706330172266920187, -0.8212051873014210024 ) ) ;
#18326=CARTESIAN_POINT ( 'NONE',  ( 43.31606138205700063, -39.23120981750657421, 69.49370132789680099 ) ) ;
#18344=DIRECTION ( 'NONE',  ( -1.000000000000000000, -6.197457809535974789E-17, -1.134781633102316229E-16 ) ) ;
#18349=FACE_OUTER_BOUND ( 'NONE', #12069, .T. ) ;
#18363=VERTEX_POINT ( 'NONE', #22770 ) ;
#18371=VERTEX_POINT ( 'NONE', #10800 ) ;
#18387=EDGE_CURVE ( 'NONE', #18958, #16794, #15425, .T. ) ;
#18390=EDGE_CURVE ( 'NONE', #20720, #1537, #20463, .T. ) ;
#18402=CARTESIAN_POINT ( 'NONE',  ( 42.90907157547642470, 3.273800194542833442, 6.355715097685992632 ) ) ;
#18408=EDGE_CURVE ( 'NONE', #21396, #6643, #13122, .T. ) ;
#18409=CARTESIAN_POINT ( 'NONE',  ( 43.31606138205700063, 4.103895195095678794, 6.341006091748962348 ) ) ;
#18416=CARTESIAN_POINT ( 'NONE',  ( 34.06606138205700773, -32.75315594507191008, 59.38245422252773409 ) ) ;
#18421=CARTESIAN_POINT ( 'NONE',  ( 43.81606138205700063, -2.088476903695762665, 19.19551655256602984 ) ) ;
#18427=DIRECTION ( 'NONE',  ( 0.000000000000000000, 0.4278636397681519488, -0.9038432971286278761 ) ) ;
#18436=CIRCLE ( 'NONE', #2369, 0.4999999999999943379 ) ;
#18437=ADVANCED_FACE ( 'NONE', ( #9647 ), #25187, .T. ) ;
#18464=ORIENTED_EDGE ( 'NONE', *, *, #109, .T. ) ;
#18478=VECTOR ( 'NONE', #17179, 1000.000000000000000 ) ;
#18482=CARTESIAN_POINT ( 'NONE',  ( 42.71151723894909225, 2.752945995551776992, 6.094624432592374852 ) ) ;
#18489=CARTESIAN_POINT ( 'NONE',  ( 33.33836326447716658, 3.869514117107255569, 6.310928887378282504 ) ) ;
#18502=LINE ( 'NONE', #20432, #25405 ) ;
#18503=CARTESIAN_POINT ( 'NONE',  ( 43.81606138205700063, -38.37466412126273951, 70.68129701848354784 ) ) ;
#18527=CARTESIAN_POINT ( 'NONE',  ( 33.77220352641053580, 2.787451151481231015, 6.090842338480662477 ) ) ;
#18540=ORIENTED_EDGE ( 'NONE', *, *, #21868, .T. ) ;
#18547=EDGE_CURVE ( 'NONE', #18363, #10132, #15678, .T. ) ;
#18571=ORIENTED_EDGE ( 'NONE', *, *, #16885, .F. ) ;
#18574=DIRECTION ( 'NONE',  ( 0.000000000000000000, -0.9911113317706403691, -0.1330350631819583740 ) ) ;
#18582=DIRECTION ( 'NONE',  ( 1.000000000000000000, 0.000000000000000000, 0.000000000000000000 ) ) ;
#18588=DIRECTION ( 'NONE',  ( 0.000000000000000000, 0.8212051873014223347, 0.5706330172266899092 ) ) ;
#18613=EDGE_CURVE ( 'NONE', #22481, #170, #2138, .T. ) ;
#18614=EDGE_CURVE ( 'NONE', #2590, #7328, #21611, .T. ) ;
#18629=VECTOR ( 'NONE', #4561, 1000.000000000000114 ) ;
#18632=DIRECTION ( 'NONE',  ( 0.000000000000000000, 0.5706330172266920187, -0.8212051873014210024 ) ) ;
#18636=VERTEX_POINT ( 'NONE', #16056 ) ;
#18639=DIRECTION ( 'NONE',  ( 0.000000000000000000, 0.5706330172266919076, -0.8212051873014208914 ) ) ;
#18648=B_SPLINE_CURVE_WITH_KNOTS ( 'NONE', 3,
 ( #6550, #12500, #18157, #8495, #14538, #8108, #10165, #21889, #4249, #18409 ),
 .UNSPECIFIED., .F., .F.,
 ( 4, 3, 3, 4 ),
 ( 2.436441354035134762E-18, 0.0001278088409237286072, 0.0002582060142820110401, 0.0003905966221991465331 ),
 .UNSPECIFIED. ) ;
#18653=LINE ( 'NONE', #18780, #6680 ) ;
#18677=DIRECTION ( 'NONE',  ( 1.000000000000000000, 1.185941393278724777E-16, 8.240782279085522416E-17 ) ) ;
#18696=EDGE_LOOP ( 'NONE', ( #7983, #16532 ) ) ;
#18722=PLANE ( 'NONE',  #9633 ) ;
#18723=CARTESIAN_POINT ( 'NONE',  ( 33.31606138205700773, -27.60498114914039647, 57.04949906928990089 ) ) ;
#18732=EDGE_CURVE ( 'NONE', #23179, #3938, #14009, .T. ) ;
#18743=FACE_OUTER_BOUND ( 'NONE', #11866, .T. ) ;
#18748=FACE_OUTER_BOUND ( 'NONE', #17826, .T. ) ;
#18751=ORIENTED_EDGE ( 'NONE', *, *, #17763, .T. ) ;
#18758=DIRECTION ( 'NONE',  ( 0.6648258951495188418, -0.6134389167572597001, -0.4262619201222657694 ) ) ;
#18765=ORIENTED_EDGE ( 'NONE', *, *, #2151, .T. ) ;
#18770=ORIENTED_EDGE ( 'NONE', *, *, #18390, .T. ) ;
#18780=CARTESIAN_POINT ( 'NONE',  ( 43.81606138205700063, -27.17722769842920272, 59.42551550655435477 ) ) ;
#18782=DIRECTION ( 'NONE',  ( 0.000000000000000000, 0.5706330172266919076, -0.8212051873014208914 ) ) ;
#18832=DIRECTION ( 'NONE',  ( 0.000000000000000000, 0.8212051873014223347, 0.5706330172266899092 ) ) ;
#18836=CARTESIAN_POINT ( 'NONE',  ( 32.81606138205700773, 6.294683054830111146, 7.131205101789720224 ) ) ;
#18848=DIRECTION ( 'NONE',  ( -1.000000000000000000, -1.187136597504755470E-16, -8.249087426255173666E-17 ) ) ;
#18856=EDGE_CURVE ( 'NONE', #16162, #18363, #18502, .T. ) ;
#18868=CARTESIAN_POINT ( 'NONE',  ( 43.78068403493972482, 3.723062046805433845, 6.249772126726830912 ) ) ;
#18918=DIRECTION ( 'NONE',  ( 0.000000000000000000, 0.8212051873014208914, 0.5706330172266919076 ) ) ;
#18919=DIRECTION ( 'NONE',  ( 1.000000000000000000, -0.000000000000000000, 0.000000000000000000 ) ) ;
#18928=AXIS2_PLACEMENT_3D ( 'NONE', #20668, #1068, #3637 ) ;
#18935=LINE ( 'NONE', #10822, #10109 ) ;
#18958=VERTEX_POINT ( 'NONE', #14657 ) ;
#18961=CARTESIAN_POINT ( 'NONE',  ( 43.81606138205700063, 7.166937456968672571, 6.752152658007350539 ) ) ;
#18980=DIRECTION ( 'NONE',  ( 1.000000000000000000, 0.000000000000000000, 0.000000000000000000 ) ) ;
#18982=DIRECTION ( 'NONE',  ( 1.000000000000000000, -0.000000000000000000, 0.000000000000000000 ) ) ;
#18991=CARTESIAN_POINT ( 'NONE',  ( 33.23058527440271348, 3.113468987225122220, 6.136968036621323286 ) ) ;
#18999=DIRECTION ( 'NONE',  ( 1.000000000000000000, -0.000000000000000000, 0.000000000000000000 ) ) ;
#19003=ADVANCED_FACE ( 'NONE', ( #999 ), #860, .T. ) ;
#19010=CARTESIAN_POINT ( 'NONE',  ( 33.88977883051490636, 3.189440311900809011, 6.370184205068262884 ) ) ;
#19020=ORIENTED_EDGE ( 'NONE', *, *, #20148, .F. ) ;
#19034=CARTESIAN_POINT ( 'NONE',  ( 42.82423818562821793, 3.225621635936315457, 6.370934609586303310 ) ) ;
#19035=VECTOR ( 'NONE', #20487, 1000.000000000000114 ) ;
#19037=EDGE_CURVE ( 'NONE', #4345, #4551, #7064, .T. ) ;
#19049=ORIENTED_EDGE ( 'NONE', *, *, #17138, .T. ) ;
#19067=DIRECTION ( 'NONE',  ( 1.000000000000000000, -0.000000000000000000, 0.000000000000000000 ) ) ;
#19086=EDGE_CURVE ( 'NONE', #21114, #1537, #5001, .T. ) ;
#19091=LINE ( 'NONE', #18961, #2070 ) ;
#19113=DIRECTION ( 'NONE',  ( -1.000000000000000000, 0.000000000000000000, 0.000000000000000000 ) ) ;
#19126=CARTESIAN_POINT ( 'NONE',  ( 43.77578593420113862, 3.724120516973108419, 6.250574242801828717 ) ) ;
#19132=EDGE_CURVE ( 'NONE', #9471, #23179, #15816, .T. ) ;
#19134=AXIS2_PLACEMENT_3D ( 'NONE', #13674, #21272, #3880 ) ;
#19144=FACE_OUTER_BOUND ( 'NONE', #14640, .T. ) ;
#19150=CARTESIAN_POINT ( 'NONE',  ( 43.52384487926482848, 3.236615080648331144, 6.150472170364783331 ) ) ;
#19158=CARTESIAN_POINT ( 'NONE',  ( 42.85805032784998758, 2.782058442729017145, 6.089052160330568952 ) ) ;
#19179=ADVANCED_FACE ( 'NONE', ( #19289 ), #11451, .F. ) ;
#19184=DIRECTION ( 'NONE',  ( 1.000000000000000000, 1.518641380243644581E-16, 1.055262346480601087E-16 ) ) ;
#19186=ADVANCED_FACE ( 'NONE', ( #1626 ), #13385, .T. ) ;
#19191=LINE ( 'NONE', #1523, #1203 ) ;
#19222=VECTOR ( 'NONE', #11496, 1000.000000000000114 ) ;
#19224=CARTESIAN_POINT ( 'NONE',  ( 43.81606138205700063, -35.70002751211045933, 71.94742330197156832 ) ) ;
#19233=EDGE_LOOP ( 'NONE', ( #6921, #21719, #13873, #7047 ) ) ;
#19242=CARTESIAN_POINT ( 'NONE',  ( 43.31606138205700063, 6.355893005198818280, 6.643287643123708008 ) ) ;
#19244=VECTOR ( 'NONE', #18049, 1000.000000000000000 ) ;
#19247=FILL_AREA_STYLE ('',( #3278 ) ) ;
#19250=EDGE_CURVE ( 'NONE', #25460, #4447, #7704, .T. ) ;
#19252=EDGE_CURVE ( 'NONE', #13033, #24417, #5520, .T. ) ;
#19257=LINE ( 'NONE', #9242, #22746 ) ;
#19260=CIRCLE ( 'NONE', #9402, 0.7500000000000006661 ) ;
#19262=DIRECTION ( 'NONE',  ( 1.000000000000000000, 0.000000000000000000, 0.000000000000000000 ) ) ;
#19264=ORIENTED_EDGE ( 'NONE', *, *, #1124, .T. ) ;
#19273=ORIENTED_EDGE ( 'NONE', *, *, #23592, .T. ) ;
#19280=DIRECTION ( 'NONE',  ( 0.000000000000000000, 0.8212051873014208914, 0.5706330172266919076 ) ) ;
#19289=FACE_OUTER_BOUND ( 'NONE', #15896, .T. ) ;
#19296=EDGE_LOOP ( 'NONE', ( #9398, #3022, #20161, #23699 ) ) ;
#19307=CARTESIAN_POINT ( 'NONE',  ( 43.31606138205700063, -20.88462213363798270, 44.49284693533410717 ) ) ;
#19324=DIRECTION ( 'NONE',  ( 0.000000000000000000, 0.5706330172266919076, -0.8212051873014208914 ) ) ;
#19328=CIRCLE ( 'NONE', #15225, 0.5000000000000011102 ) ;
#19336=LINE ( 'NONE', #9693, #19222 ) ;
#19337=ORIENTED_EDGE ( 'NONE', *, *, #8169, .F. ) ;
#19339=DIRECTION ( 'NONE',  ( 0.000000000000000000, 0.8212051873014208914, 0.5706330172266919076 ) ) ;
#19347=EDGE_CURVE ( 'NONE', #21396, #20637, #22111, .T. ) ;
#19353=FACE_OUTER_BOUND ( 'NONE', #3728, .T. ) ;
#19376=CARTESIAN_POINT ( 'NONE',  ( 40.56606138205700773, 5.594015759443068170, 2.006005027196319901 ) ) ;
#19380=DIRECTION ( 'NONE',  ( -0.000000000000000000, -0.1330350631819583740, 0.9911113317706403691 ) ) ;
#19387=CARTESIAN_POINT ( 'NONE',  ( 33.31606138205700773, 6.705285648480822758, 7.416521610403067122 ) ) ;
#19409=CARTESIAN_POINT ( 'NONE',  ( 43.39391466435857581, 3.105264735554318811, 6.136852473770198380 ) ) ;
#19418=ORIENTED_EDGE ( 'NONE', *, *, #24621, .F. ) ;
#19426=CARTESIAN_POINT ( 'NONE',  ( 33.63430007298546087, 2.841684771932709186, 6.101742786271089791 ) ) ;
#19432=DIRECTION ( 'NONE',  ( -1.000000000000000000, 0.000000000000000000, 0.000000000000000000 ) ) ;
#19459=ADVANCED_FACE ( 'NONE', ( #6154, #16060 ), #2519, .F. ) ;
#19466=DIRECTION ( 'NONE',  ( -1.000000000000000000, 0.000000000000000000, 0.000000000000000000 ) ) ;
#19471=AXIS2_PLACEMENT_3D ( 'NONE', #22456, #22840, #18848 ) ;
#19476=CARTESIAN_POINT ( 'NONE',  ( 40.81606138205700773, -29.78523130861184143, 52.92072663988442116 ) ) ;
#19488=ORIENTED_EDGE ( 'NONE', *, *, #25429, .F. ) ;
#19500=CARTESIAN_POINT ( 'NONE',  ( 43.31606138205700063, 7.166937456968672571, 6.752152658007350539 ) ) ;
#19504=DIRECTION ( 'NONE',  ( 0.000000000000000000, -0.5706330172266907974, 0.8212051873014217795 ) ) ;
#19519=AXIS2_PLACEMENT_3D ( 'NONE', #9977, #9477, #4175 ) ;
#19539=CARTESIAN_POINT ( 'NONE',  ( 42.82341778883947825, 3.225255403573667135, 6.370938332379879832 ) ) ;
#19542=ORIENTED_EDGE ( 'NONE', *, *, #10888, .T. ) ;
#19545=DIRECTION ( 'NONE',  ( 0.000000000000000000, -0.8212051873014203363, -0.5706330172266926848 ) ) ;
#19547=CARTESIAN_POINT ( 'NONE',  ( 40.56606138205700773, 5.719301844480432884, 2.701924129460374413 ) ) ;
#19555=VERTEX_POINT ( 'NONE', #24527 ) ;
#19561=VERTEX_POINT ( 'NONE', #16953 ) ;
#19566=LINE ( 'NONE', #15448, #20138 ) ;
#19590=ORIENTED_EDGE ( 'NONE', *, *, #7843, .F. ) ;
#19594=CARTESIAN_POINT ( 'NONE',  ( 33.31606138205700773, -21.50052602411404834, 44.06487217241408416 ) ) ;
#19619=DIRECTION ( 'NONE',  ( -1.000000000000000000, 0.000000000000000000, 0.000000000000000000 ) ) ;
#19626=EDGE_CURVE ( 'NONE', #16259, #4087, #13318, .T. ) ;
#19630=CARTESIAN_POINT ( 'NONE',  ( 33.35284519649047752, 2.993954861727095906, 6.108562081104513375 ) ) ;
#19632=FACE_OUTER_BOUND ( 'NONE', #12282, .T. ) ;
#19655=ORIENTED_EDGE ( 'NONE', *, *, #3018, .F. ) ;
#19683=VERTEX_POINT ( 'NONE', #25033 ) ;
#19727=LINE ( 'NONE', #514, #24141 ) ;
#19739=VECTOR ( 'NONE', #16595, 1000.000000000000114 ) ;
#19760=ORIENTED_EDGE ( 'NONE', *, *, #20314, .F. ) ;
#19768=VECTOR ( 'NONE', #8154, 1000.000000000000114 ) ;
#19775=EDGE_LOOP ( 'NONE', ( #12334, #23423, #13332, #1893 ) ) ;
#19784=VERTEX_POINT ( 'NONE', #23245 ) ;
#19789=DIRECTION ( 'NONE',  ( 0.000000000000000000, -0.8212051873014252212, -0.5706330172266858014 ) ) ;
#19794=DIRECTION ( 'NONE',  ( 1.000000000000000000, -0.000000000000000000, 0.000000000000000000 ) ) ;
#19812=ORIENTED_EDGE ( 'NONE', *, *, #19132, .F. ) ;
#19822=ORIENTED_EDGE ( 'NONE', *, *, #8560, .F. ) ;
#19826=DIRECTION ( 'NONE',  ( 0.000000000000000000, 0.5706330172266952383, -0.8212051873014186709 ) ) ;
#19830=PLANE ( 'NONE',  #24208 ) ;
#19839=VERTEX_POINT ( 'NONE', #23875 ) ;
#19840=ORIENTED_EDGE ( 'NONE', *, *, #9662, .F. ) ;
#19844=DIRECTION ( 'NONE',  ( -1.000000000000000000, 0.000000000000000000, 0.000000000000000000 ) ) ;
#19854=CARTESIAN_POINT ( 'NONE',  ( 33.24019963865212191, 3.104051971978903701, 6.135536383744724098 ) ) ;
#19881=VERTEX_POINT ( 'NONE', #4056 ) ;
#19888=AXIS2_PLACEMENT_3D ( 'NONE', #5447, #1321, #1449 ) ;
#19904=CARTESIAN_POINT ( 'NONE',  ( 33.31606138205700773, -20.88462213363798270, 44.49284693533410717 ) ) ;
#19916=ORIENTED_EDGE ( 'NONE', *, *, #12714, .T. ) ;
#19921=DIRECTION ( 'NONE',  ( 0.000000000000000000, -0.5706330172266919076, 0.8212051873014208914 ) ) ;
#19936=CARTESIAN_POINT ( 'NONE',  ( 33.31606138205700773, 3.172506336381830661, 12.50058896911730066 ) ) ;
#19940=VERTEX_POINT ( 'NONE', #9988 ) ;
#19943=PLANE ( 'NONE',  #21891 ) ;
#19949=AXIS2_PLACEMENT_3D ( 'NONE', #3180, #6930, #6803 ) ;
#19953=CARTESIAN_POINT ( 'NONE',  ( 43.13775064171697693, 2.905199411292878953, 6.099582584402872598 ) ) ;
#19954=CARTESIAN_POINT ( 'NONE',  ( 43.81606138205700063, -37.34243788671330577, 70.80615726751818784 ) ) ;
#19960=CARTESIAN_POINT ( 'NONE',  ( 43.81606138205700063, -21.31259689655800216, 45.10875082581016926 ) ) ;
#19962=CARTESIAN_POINT ( 'NONE',  ( 43.05893433410182070, 3.408565912792066221, 6.350990188909392486 ) ) ;
#19980=DIRECTION ( 'NONE',  ( 0.000000000000000000, -0.5706330172266952383, 0.8212051873014186709 ) ) ;
#19983=FACE_OUTER_BOUND ( 'NONE', #12403, .T. ) ;
#20004=VERTEX_POINT ( 'NONE', #2994 ) ;
#20008=B_SPLINE_CURVE_WITH_KNOTS ( 'NONE', 3,
 ( #20037, #16415, #18489, #22223, #22092, #2877 ),
 .UNSPECIFIED., .F., .F.,
 ( 4, 2, 4 ),
 ( 0.000000000000000000, 0.5000000000000000000, 1.000000000000000000 ),
 .UNSPECIFIED. ) ;
#20009=DIRECTION ( 'NONE',  ( 1.000000000000000000, 1.187136597504755470E-16, 8.249087426255173666E-17 ) ) ;
#20017=CARTESIAN_POINT ( 'NONE',  ( 33.23689862680489426, 3.100967383408606448, 6.133394271278472587 ) ) ;
#20022=ORIENTED_EDGE ( 'NONE', *, *, #10523, .T. ) ;
#20026=CARTESIAN_POINT ( 'NONE',  ( 43.31606138205700063, -33.70281195181703993, 69.07320514641659770 ) ) ;
#20027=ORIENTED_EDGE ( 'NONE', *, *, #18033, .F. ) ;
#20030=ORIENTED_EDGE ( 'NONE', *, *, #554, .T. ) ;
#20037=CARTESIAN_POINT ( 'NONE',  ( 33.31606138205700773, 4.124002793203064066, 6.312068993173404863 ) ) ;
#20049=EDGE_LOOP ( 'NONE', ( #12847, #15458, #11556, #21206 ) ) ;
#20059=VECTOR ( 'NONE', #1044, 1000.000000000000000 ) ;
#20060=DIRECTION ( 'NONE',  ( 1.000000000000000000, -0.000000000000000000, 0.000000000000000000 ) ) ;
#20063=VECTOR ( 'NONE', #23666, 1000.000000000000114 ) ;
#20066=ORIENTED_EDGE ( 'NONE', *, *, #5941, .F. ) ;
#20086=LINE ( 'NONE', #20467, #19739 ) ;
#20097=CARTESIAN_POINT ( 'NONE',  ( 32.81606138205700773, -36.11063010576116739, 71.66210679335823386 ) ) ;
#20098=EDGE_CURVE ( 'NONE', #11457, #5208, #12438, .T. ) ;
#20107=CARTESIAN_POINT ( 'NONE',  ( 43.81608638205700146, 2.887189827768484207, 12.91119156276801228 ) ) ;
#20116=CARTESIAN_POINT ( 'NONE',  ( 43.18074167159075216, 3.582118287471805385, 6.336670741225087333 ) ) ;
#20138=VECTOR ( 'NONE', #23292, 1000.000000000000114 ) ;
#20140=LINE ( 'NONE', #24108, #7189 ) ;
#20148=EDGE_CURVE ( 'NONE', #20521, #952, #22334, .T. ) ;
#20161=ORIENTED_EDGE ( 'NONE', *, *, #21086, .F. ) ;
#20170=ORIENTED_EDGE ( 'NONE', *, *, #16974, .F. ) ;
#20193=EDGE_LOOP ( 'NONE', ( #4344, #20702, #689, #21056 ) ) ;
#20202=VECTOR ( 'NONE', #21204, 1000.000000000000000 ) ;
#20217=DIRECTION ( 'NONE',  ( -1.000000000000000000, 0.000000000000000000, 0.000000000000000000 ) ) ;
#20231=CARTESIAN_POINT ( 'NONE',  ( 33.31606138205700773, -20.88462213363798270, 44.49284693533410717 ) ) ;
#20232=DIRECTION ( 'NONE',  ( 0.000000000000000000, 0.5706330172266907974, -0.8212051873014217795 ) ) ;
#20242=CARTESIAN_POINT ( 'NONE',  ( 38.31606138205700063, -29.37462871496113337, 53.20604314849776983 ) ) ;
#20269=ORIENTED_EDGE ( 'NONE', *, *, #16116, .T. ) ;
#20270=CARTESIAN_POINT ( 'NONE',  ( 34.06606138205700773, -33.77966242919868733, 58.66916295099436951 ) ) ;
#20298=EDGE_LOOP ( 'NONE', ( #4822, #20022, #5336, #22930 ) ) ;
#20302=EDGE_CURVE ( 'NONE', #2134, #10314, #1191, .T. ) ;
#20305=EDGE_CURVE ( 'NONE', #24159, #14544, #7643, .T. ) ;
#20314=EDGE_CURVE ( 'NONE', #10213, #9175, #7258, .T. ) ;
#20330=ORIENTED_EDGE ( 'NONE', *, *, #24621, .T. ) ;
#20338=ADVANCED_FACE ( 'NONE', ( #9080 ), #25126, .T. ) ;
#20340=FACE_OUTER_BOUND ( 'NONE', #17335, .T. ) ;
#20346=ORIENTED_EDGE ( 'NONE', *, *, #7148, .F. ) ;
#20348=MECHANICAL_DESIGN_GEOMETRIC_PRESENTATION_REPRESENTATION('',(#8422),#21988);
#20350=ORIENTED_EDGE ( 'NONE', *, *, #25128, .F. ) ;
#20362=LINE ( 'NONE', #12144, #16456 ) ;
#20372=CARTESIAN_POINT ( 'NONE',  ( 33.80700705136447937, 3.227014435054107455, 6.369498925975481285 ) ) ;
#20377=LINE ( 'NONE', #2584, #9773 ) ;
#20383=CARTESIAN_POINT ( 'NONE',  ( 42.82259792697934841, 3.224889410007908630, 6.370942052746025652 ) ) ;
#20428=ORIENTED_EDGE ( 'NONE', *, *, #13490, .T. ) ;
#20432=CARTESIAN_POINT ( 'NONE',  ( 40.56606138205700773, 2.740850673309605412, 6.112030963703427133 ) ) ;
#20442=AXIS2_PLACEMENT_3D ( 'NONE', #20551, #20681, #22862 ) ;
#20446=CIRCLE ( 'NONE', #1103, 0.7500000000000031086 ) ;
#20457=CARTESIAN_POINT ( 'NONE',  ( 32.81606138205700773, -27.52349462642295208, 56.67559192035834315 ) ) ;
#20462=VECTOR ( 'NONE', #24206, 1000.000000000000114 ) ;
#20463=CIRCLE ( 'NONE', #1946, 0.5000000000000004441 ) ;
#20467=CARTESIAN_POINT ( 'NONE',  ( 32.81606138205700773, -37.34243788671330577, 70.80615726751818784 ) ) ;
#20468=DIRECTION ( 'NONE',  ( 0.000000000000000000, -0.8212051873014297732, -0.5706330172266793621 ) ) ;
#20470=ORIENTED_EDGE ( 'NONE', *, *, #18614, .F. ) ;
#20475=AXIS2_PLACEMENT_3D ( 'NONE', #19376, #23626, #5983 ) ;
#20487=DIRECTION ( 'NONE',  ( 6.938893903907229364E-16, 0.8212051873014208914, 0.5706330172266919076 ) ) ;
#20494=VECTOR ( 'NONE', #21865, 1000.000000000000114 ) ;
#20495=ORIENTED_EDGE ( 'NONE', *, *, #25058, .F. ) ;
#20504=ORIENTED_EDGE ( 'NONE', *, *, #10564, .T. ) ;
#20511=ORIENTED_EDGE ( 'NONE', *, *, #22406, .F. ) ;
#20521=VERTEX_POINT ( 'NONE', #11894 ) ;
#20523=DIRECTION ( 'NONE',  ( 0.000000000000000000, -0.5706330172266919076, 0.8212051873014208914 ) ) ;
#20529=DIRECTION ( 'NONE',  ( 0.000000000000000000, -0.8212051873014210024, -0.5706330172266920187 ) ) ;
#20551=CARTESIAN_POINT ( 'NONE',  ( 38.31606138205700063, -6.959910619544160681, 20.07251914782758107 ) ) ;
#20566=EDGE_CURVE ( 'NONE', #8460, #5709, #23717, .T. ) ;
#20622=EDGE_CURVE ( 'NONE', #3766, #19561, #7742, .T. ) ;
#20637=VERTEX_POINT ( 'NONE', #2580 ) ;
#20649=EDGE_CURVE ( 'NONE', #2026, #25158, #11926, .T. ) ;
#20668=CARTESIAN_POINT ( 'NONE',  ( 43.81606138205700063, -2.373793412309109563, 19.60611914621674146 ) ) ;
#20681=DIRECTION ( 'NONE',  ( -1.849283715844614702E-16, 0.8212051873014210024, 0.5706330172266920187 ) ) ;
#20690=AXIS2_PLACEMENT_3D ( 'NONE', #8360, #13896, #21752 ) ;
#20702=ORIENTED_EDGE ( 'NONE', *, *, #14232, .T. ) ;
#20704=CARTESIAN_POINT ( 'NONE',  ( 32.81606138205700773, -3.566646240838321269, 18.16837712155798457 ) ) ;
#20720=VERTEX_POINT ( 'NONE', #897 ) ;
#20725=CARTESIAN_POINT ( 'NONE',  ( 33.31606138205700773, -33.60910547091194900, 60.61426200347987248 ) ) ;
#20726=DIRECTION ( 'NONE',  ( 1.000000000000000000, 7.979170143241514824E-17, -1.148292460158762122E-16 ) ) ;
#20733=ORIENTED_EDGE ( 'NONE', *, *, #15389, .T. ) ;
#20744=EDGE_LOOP ( 'NONE', ( #23795, #22498, #10151, #15446 ) ) ;
#20748=DIRECTION ( 'NONE',  ( -1.000000000000000000, 0.000000000000000000, 0.000000000000000000 ) ) ;
#20752=AXIS2_PLACEMENT_3D ( 'NONE', #3136, #15117, #24630 ) ;
#20775=EDGE_CURVE ( 'NONE', #6643, #12177, #3600, .T. ) ;
#20796=LINE ( 'NONE', #1194, #16329 ) ;
#20805=EDGE_CURVE ( 'NONE', #16606, #23317, #1595, .T. ) ;
#20815=VERTEX_POINT ( 'NONE', #7096 ) ;
#20822=CARTESIAN_POINT ( 'NONE',  ( 43.13768477939176194, 2.905169009495293331, 6.099583767035779758 ) ) ;
#20826=CARTESIAN_POINT ( 'NONE',  ( 43.81606138205700063, -37.81581049437287589, 70.47722359350073873 ) ) ;
#20827=ORIENTED_EDGE ( 'NONE', *, *, #15560, .F. ) ;
#20834=ORIENTED_EDGE ( 'NONE', *, *, #15258, .F. ) ;
#20848=CARTESIAN_POINT ( 'NONE',  ( 43.63145769492233228, 3.383950488897877307, 6.176937329184648995 ) ) ;
#20852=DIRECTION ( 'NONE',  ( 0.000000000000000000, -0.5706330172266952383, 0.8212051873014186709 ) ) ;
#20866=EDGE_LOOP ( 'NONE', ( #20170, #20511 ) ) ;
#20875=DIRECTION ( 'NONE',  ( -0.6606874543841287917, -0.6164467895351006810, -0.4283520086229165025 ) ) ;
#20898=LINE ( 'NONE', #5433, #22001 ) ;
#20902=DIRECTION ( 'NONE',  ( 0.000000000000000000, -0.8212051873014213355, -0.5706330172266915746 ) ) ;
#20911=DIRECTION ( 'NONE',  ( 1.000000000000000000, 0.000000000000000000, 0.000000000000000000 ) ) ;
#20955=EDGE_LOOP ( 'NONE', ( #16473, #21642, #10062, #7213 ) ) ;
#20963=ORIENTED_EDGE ( 'NONE', *, *, #4964, .T. ) ;
#20983=ORIENTED_EDGE ( 'NONE', *, *, #18732, .T. ) ;
#20987=ORIENTED_EDGE ( 'NONE', *, *, #16304, .F. ) ;
#21013=EDGE_LOOP ( 'NONE', ( #15016, #2643 ) ) ;
#21019=B_SPLINE_SURFACE_WITH_KNOTS ( 'NONE', 1, 3, ( 
 ( #20017, #19630, #6109, #9855 ),
 ( #43, #17714, #18098, #2355 ),
 ( #23992, #7924, #6370, #12301 ) ),
 .UNSPECIFIED., .F., .F., .F.,
 ( 2, 1, 2 ),
 ( 4, 4 ),
 ( -0.01000000000000000021, 0.000000000000000000, 1.000000000000000000 ),
 ( 0.000000000000000000, 1.000000000000000000 ),
 .UNSPECIFIED. ) ;
#21026=EDGE_LOOP ( 'NONE', ( #2053, #17351, #9637, #7920 ) ) ;
#21035=CARTESIAN_POINT ( 'NONE',  ( 43.31606138205700063, -20.45664737071796324, 43.87694304485803798 ) ) ;
#21041=FACE_OUTER_BOUND ( 'NONE', #5229, .T. ) ;
#21050=ORIENTED_EDGE ( 'NONE', *, *, #7275, .F. ) ;
#21056=ORIENTED_EDGE ( 'NONE', *, *, #4286, .F. ) ;
#21060=ORIENTED_EDGE ( 'NONE', *, *, #4286, .T. ) ;
#21067=EDGE_CURVE ( 'NONE', #23614, #22308, #20086, .T. ) ;
#21086=EDGE_CURVE ( 'NONE', #9087, #12177, #8224, .T. ) ;
#21090=ORIENTED_EDGE ( 'NONE', *, *, #5941, .T. ) ;
#21098=VECTOR ( 'NONE', #13524, 1000.000000000000000 ) ;
#21106=DIRECTION ( 'NONE',  ( 1.022195611122249672E-16, -0.1771812806364704007, -0.9841782327363373106 ) ) ;
#21110=CARTESIAN_POINT ( 'NONE',  ( 33.31606138205700773, -27.52349462642295208, 56.67559192035834315 ) ) ;
#21114=VERTEX_POINT ( 'NONE', #21110 ) ;
#21146=ORIENTED_EDGE ( 'NONE', *, *, #7061, .T. ) ;
#21147=DIRECTION ( 'NONE',  ( -1.849283715844614702E-16, 0.8212051873014210024, 0.5706330172266920187 ) ) ;
#21171=CARTESIAN_POINT ( 'NONE',  ( 43.81606138205700063, 3.172506336381830661, 12.50058896911730066 ) ) ;
#21194=ORIENTED_EDGE ( 'NONE', *, *, #22369, .F. ) ;
#21198=DIRECTION ( 'NONE',  ( 0.000000000000000000, 0.5706330172266952383, -0.8212051873014186709 ) ) ;
#21204=DIRECTION ( 'NONE',  ( -1.000000000000000000, -1.159780179694326360E-16, -8.617271610285116919E-17 ) ) ;
#21206=ORIENTED_EDGE ( 'NONE', *, *, #10888, .F. ) ;
#21221=CARTESIAN_POINT ( 'NONE',  ( 42.99772342963552774, 2.840642293467601665, 6.103164780676344492 ) ) ;
#21256=CARTESIAN_POINT ( 'NONE',  ( 32.81606138205700773, -37.53049398575952722, 70.06662099985001646 ) ) ;
#21272=DIRECTION ( 'NONE',  ( -1.000000000000000000, -1.187136597504755470E-16, -8.249087426255172434E-17 ) ) ;
#21275=CARTESIAN_POINT ( 'NONE',  ( 33.31606138205700773, -39.60075215179220720, 69.23691647014479145 ) ) ;
#21283=PRODUCT_CONTEXT ( 'NONE', #15728, 'mechanical' ) ;
#21285=CARTESIAN_POINT ( 'NONE',  ( 32.81106138205699807, 4.124002793203064066, 6.312068993173404863 ) ) ;
#21347=EDGE_CURVE ( 'NONE', #19881, #4087, #6380, .T. ) ;
#21351=CIRCLE ( 'NONE', #4893, 2.500000000000002220 ) ;
#21356=ORIENTED_EDGE ( 'NONE', *, *, #12099, .T. ) ;
#21380=EDGE_CURVE ( 'NONE', #11138, #16259, #21707, .T. ) ;
#21391=AXIS2_PLACEMENT_3D ( 'NONE', #17853, #21831, #2110 ) ;
#21396=VERTEX_POINT ( 'NONE', #20026 ) ;
#21422=ORIENTED_EDGE ( 'NONE', *, *, #15856, .T. ) ;
#21425=CARTESIAN_POINT ( 'NONE',  ( 43.30090830489194786, -32.87633672316712108, 59.29685926994373091 ) ) ;
#21436=EDGE_CURVE ( 'NONE', #9471, #24226, #24624, .T. ) ;
#21446=SHAPE_REPRESENTATION_RELATIONSHIP ( 'NONE' , 'NONE' ,  #14587, #24269 ) ;
#21449=ORIENTED_EDGE ( 'NONE', *, *, #20649, .T. ) ;
#21465=LINE ( 'NONE', #21721, #13691 ) ;
#21471=FACE_OUTER_BOUND ( 'NONE', #20193, .T. ) ;
#21475=ORIENTED_EDGE ( 'NONE', *, *, #14939, .F. ) ;
#21476=FACE_OUTER_BOUND ( 'NONE', #18103, .T. ) ;
#21479=DIRECTION ( 'NONE',  ( 1.000000000000000000, -0.000000000000000000, 0.000000000000000000 ) ) ;
#21483=VECTOR ( 'NONE', #19280, 1000.000000000000114 ) ;
#21508=EDGE_CURVE ( 'NONE', #170, #13976, #20796, .T. ) ;
#21513=ORIENTED_EDGE ( 'NONE', *, *, #2938, .T. ) ;
#21530=ORIENTED_EDGE ( 'NONE', *, *, #20314, .T. ) ;
#21532=FACE_OUTER_BOUND ( 'NONE', #8183, .T. ) ;
#21538=CARTESIAN_POINT ( 'NONE',  ( 43.31606138205700063, -27.60498114914042134, 57.04949906928993641 ) ) ;
#21548=CARTESIAN_POINT ( 'NONE',  ( 43.23188216675521289, 3.685658823189455369, 6.335155785894674096 ) ) ;
#21574=DIRECTION ( 'NONE',  ( -1.000000000000000000, 0.000000000000000000, 0.000000000000000000 ) ) ;
#21579=( LENGTH_UNIT ( ) NAMED_UNIT ( * ) SI_UNIT ( .MILLI., .METRE. ) );
#21585=CARTESIAN_POINT ( 'NONE',  ( 43.24580177837434292, 3.721690752961227755, 6.335617458560805382 ) ) ;
#21596=EDGE_LOOP ( 'NONE', ( #21708, #16309, #22880, #22600 ) ) ;
#21607=ORIENTED_EDGE ( 'NONE', *, *, #18387, .F. ) ;
#21611=LINE ( 'NONE', #7830, #2375 ) ;
#21612=CARTESIAN_POINT ( 'NONE',  ( 34.06606138205700773, 2.740850673309605412, 6.112030963703427133 ) ) ;
#21642=ORIENTED_EDGE ( 'NONE', *, *, #22369, .T. ) ;
#21644=VECTOR ( 'NONE', #8905, 1000.000000000000000 ) ;
#21669=EDGE_CURVE ( 'NONE', #17745, #19683, #5243, .T. ) ;
#21670=AXIS2_PLACEMENT_3D ( 'NONE', #11552, #23248, #19262 ) ;
#21697=DIRECTION ( 'NONE',  ( -1.000000000000000000, -1.187136597504755470E-16, -8.249087426255173666E-17 ) ) ;
#21707=LINE ( 'NONE', #182, #14680 ) ;
#21708=ORIENTED_EDGE ( 'NONE', *, *, #3412, .F. ) ;
#21719=ORIENTED_EDGE ( 'NONE', *, *, #10364, .T. ) ;
#21720=DIRECTION ( 'NONE',  ( 0.000000000000000000, -0.5706330172266919076, 0.8212051873014208914 ) ) ;
#21721=CARTESIAN_POINT ( 'NONE',  ( 33.31606138205700773, -27.52349462642295208, 56.67559192035834315 ) ) ;
#21736=AXIS2_PLACEMENT_3D ( 'NONE', #17627, #13254, #15170 ) ;
#21739=DIRECTION ( 'NONE',  ( 1.000000000000000000, 1.185941393278724777E-16, 8.240782279085522416E-17 ) ) ;
#21752=DIRECTION ( 'NONE',  ( -1.000000000000000000, 0.000000000000000000, 0.000000000000000000 ) ) ;
#21758=FACE_OUTER_BOUND ( 'NONE', #24043, .T. ) ;
#21764=CARTESIAN_POINT ( 'NONE',  ( 33.31606138205700773, -40.62725863591898445, 68.52362519861142687 ) ) ;
#21770=ADVANCED_FACE ( 'NONE', ( #18196 ), #7901, .T. ) ;
#21787=DIRECTION ( 'NONE',  ( -1.000000000000000000, -7.497642437004238434E-16, 3.111695294957277996E-17 ) ) ;
#21788=VECTOR ( 'NONE', #25094, 1000.000000000000114 ) ;
#21796=FACE_OUTER_BOUND ( 'NONE', #9189, .T. ) ;
#21806=ORIENTED_EDGE ( 'NONE', *, *, #13047, .F. ) ;
#21808=CARTESIAN_POINT ( 'NONE',  ( 32.81606138205700773, -2.088476903695762665, 19.19551655256602984 ) ) ;
#21818=ORIENTED_EDGE ( 'NONE', *, *, #17196, .F. ) ;
#21827=AXIS2_PLACEMENT_3D ( 'NONE', #3681, #17606, #13862 ) ;
#21831=DIRECTION ( 'NONE',  ( -1.000000000000000000, 0.000000000000000000, 0.000000000000000000 ) ) ;
#21842=ORIENTED_EDGE ( 'NONE', *, *, #4833, .T. ) ;
#21854=EDGE_CURVE ( 'NONE', #2100, #14645, #20446, .T. ) ;
#21862=CARTESIAN_POINT ( 'NONE',  ( 33.31606138205700773, -32.95845724189726411, 59.23979596822106686 ) ) ;
#21865=DIRECTION ( 'NONE',  ( 0.000000000000000000, 0.5706330172266919076, -0.8212051873014208914 ) ) ;
#21868=EDGE_CURVE ( 'NONE', #23317, #25393, #20377, .T. ) ;
#21875=FACE_OUTER_BOUND ( 'NONE', #24418, .T. ) ;
#21878=EDGE_CURVE ( 'NONE', #13976, #3066, #12658, .T. ) ;
#21885=CARTESIAN_POINT ( 'NONE',  ( 42.82259773799690805, 3.224889347397511763, 6.370942022298698326 ) ) ;
#21889=CARTESIAN_POINT ( 'NONE',  ( 43.31331964531621281, 4.015598734371947032, 6.338464250156571111 ) ) ;
#21891=AXIS2_PLACEMENT_3D ( 'NONE', #22121, #469, #10155 ) ;
#21893=DIRECTION ( 'NONE',  ( -1.000000000000000000, -1.187136597504755470E-16, -8.249087426255172434E-17 ) ) ;
#21895=EDGE_LOOP ( 'NONE', ( #10237, #6381, #798, #24132 ) ) ;
#21903=DIRECTION ( 'NONE',  ( -1.000000000000000000, 0.000000000000000000, 0.000000000000000000 ) ) ;
#21908=VECTOR ( 'NONE', #6258, 1000.000000000000114 ) ;
#21988=( GEOMETRIC_REPRESENTATION_CONTEXT ( 3 ) GLOBAL_UNCERTAINTY_ASSIGNED_CONTEXT ( ( #4069 ) ) GLOBAL_UNIT_ASSIGNED_CONTEXT ( ( #4040, #17324, #17577 ) ) REPRESENTATION_CONTEXT ( 'NONE', 'WORKASPACE' ) );
#22001=VECTOR ( 'NONE', #9318, 1000.000000000000000 ) ;
#22006=VERTEX_POINT ( 'NONE', #1159 ) ;
#22033=DIRECTION ( 'NONE',  ( -1.000000000000000000, 0.000000000000000000, 0.000000000000000000 ) ) ;
#22051=ORIENTED_EDGE ( 'NONE', *, *, #13196, .F. ) ;
#22058=ORIENTED_EDGE ( 'NONE', *, *, #23592, .F. ) ;
#22069=DIRECTION ( 'NONE',  ( 0.000000000000000000, -0.5706330172267045642, 0.8212051873014122316 ) ) ;
#22075=ORIENTED_EDGE ( 'NONE', *, *, #23237, .T. ) ;
#22082=CARTESIAN_POINT ( 'NONE',  ( 35.81606138205700063, -29.78523130861184498, 52.92072663988442116 ) ) ;
#22092=CARTESIAN_POINT ( 'NONE',  ( 33.48677699869404023, 3.517612739349352591, 6.329933951274631099 ) ) ;
#22095=CARTESIAN_POINT ( 'NONE',  ( 43.31606138205700063, -2.088476903695762665, 19.19551655256602984 ) ) ;
#22104=VERTEX_POINT ( 'NONE', #6311 ) ;
#22111=LINE ( 'NONE', #11835, #20494 ) ;
#22117=ADVANCED_FACE ( 'NONE', ( #24181 ), #10054, .F. ) ;
#22121=CARTESIAN_POINT ( 'NONE',  ( 32.81606138205700773, -37.34243788671330577, 70.80615726751818784 ) ) ;
#22136=DIRECTION ( 'NONE',  ( -1.000000000000000000, 0.000000000000000000, 0.000000000000000000 ) ) ;
#22140=ORIENTED_EDGE ( 'NONE', *, *, #21347, .T. ) ;
#22142=ADVANCED_FACE ( 'NONE', ( #18038, #8497 ), #8241, .F. ) ;
#22150=VECTOR ( 'NONE', #354, 1000.000000000000000 ) ;
#22188=ADVANCED_FACE ( 'NONE', ( #10430 ), #2549, .F. ) ;
#22191=CARTESIAN_POINT ( 'NONE',  ( 33.31606138205700773, -30.89740888249930961, 1.247106086993583718 ) ) ;
#22193=CARTESIAN_POINT ( 'NONE',  ( 32.82453668393288382, -33.17626737717533558, 59.69730689378931032 ) ) ;
#22196=ORIENTED_EDGE ( 'NONE', *, *, #4054, .F. ) ;
#22222=ORIENTED_EDGE ( 'NONE', *, *, #8040, .F. ) ;
#22223=CARTESIAN_POINT ( 'NONE',  ( 33.42374909935192306, 3.629904212211158221, 6.320127632620215152 ) ) ;
#22233=CARTESIAN_POINT ( 'NONE',  ( 42.56606138205700063, 2.740850673309605412, 6.112030963703427133 ) ) ;
#22242=CARTESIAN_POINT ( 'NONE',  ( 43.31606138205700063, -27.66931681479738003, 59.51410614687260647 ) ) ;
#22249=EDGE_CURVE ( 'NONE', #25460, #17088, #14540, .T. ) ;
#22253=ORIENTED_EDGE ( 'NONE', *, *, #4052, .F. ) ;
#22261=CARTESIAN_POINT ( 'NONE',  ( 34.06606138205700773, -37.53049398575952722, 70.06662099985001646 ) ) ;
#22270=AXIS2_PLACEMENT_3D ( 'NONE', #11761, #23455, #7497 ) ;
#22288=ADVANCED_FACE ( 'NONE', ( #22522 ), #16593, .T. ) ;
#22308=VERTEX_POINT ( 'NONE', #14915 ) ;
#22315=ORIENTED_EDGE ( 'NONE', *, *, #9784, .T. ) ;
#22334=LINE ( 'NONE', #24246, #11906 ) ;
#22336=CARTESIAN_POINT ( 'NONE',  ( 32.81606138205700773, -37.81581049437288300, 70.47722359350072452 ) ) ;
#22369=EDGE_CURVE ( 'NONE', #17597, #13983, #9143, .T. ) ;
#22379=STYLED_ITEM ( 'NONE', ( #3928 ), #24269 ) ;
#22406=EDGE_CURVE ( 'NONE', #16742, #3435, #15990, .T. ) ;
#22410=VERTEX_POINT ( 'NONE', #1392 ) ;
#22414=VERTEX_POINT ( 'NONE', #11331 ) ;
#22430=DIRECTION ( 'NONE',  ( -1.445602896647339656E-16, 0.8212051873014208914, 0.5706330172266919076 ) ) ;
#22436=LINE ( 'NONE', #24862, #16883 ) ;
#22442=CARTESIAN_POINT ( 'NONE',  ( 34.06606138205700773, -40.21665604226827639, 68.80894170722476133 ) ) ;
#22456=CARTESIAN_POINT ( 'NONE',  ( 43.81608638205700146, -3.566646240838321269, 18.16837712155798457 ) ) ;
#22457=EDGE_CURVE ( 'NONE', #19683, #17745, #21351, .T. ) ;
#22468=B_SPLINE_CURVE_WITH_KNOTS ( 'NONE', 3,
 ( #5090, #19126, #10890, #5344 ),
 .UNSPECIFIED., .F., .F.,
 ( 4, 4 ),
 ( 0.000000000000000000, 1.000000000000000000 ),
 .UNSPECIFIED. ) ;
#22481=VERTEX_POINT ( 'NONE', #1628 ) ;
#22489=FACE_OUTER_BOUND ( 'NONE', #530, .T. ) ;
#22498=ORIENTED_EDGE ( 'NONE', *, *, #17489, .T. ) ;
#22510=CARTESIAN_POINT ( 'NONE',  ( 43.31606138205700063, -10.80800258567212602, 32.62011605800211811 ) ) ;
#22517=CARTESIAN_POINT ( 'NONE',  ( 43.81606138205700063, -27.52349462642295208, 56.67559192035834315 ) ) ;
#22518=VECTOR ( 'NONE', #1682, 1000.000000000000114 ) ;
#22521=DIRECTION ( 'NONE',  ( 4.584595141645219056E-18, 0.5706330172266919076, -0.8212051873014208914 ) ) ;
#22522=FACE_OUTER_BOUND ( 'NONE', #6418, .T. ) ;
#22537=DIRECTION ( 'NONE',  ( 1.000000000000000000, 0.000000000000000000, 0.000000000000000000 ) ) ;
#22555=VERTEX_POINT ( 'NONE', #5902 ) ;
#22569=DIRECTION ( 'NONE',  ( 0.000000000000000000, 0.5706330172266919076, -0.8212051873014208914 ) ) ;
#22571=DIRECTION ( 'NONE',  ( 1.000000000000000000, 1.518641380243644581E-16, 1.055262346480601087E-16 ) ) ;
#22579=PLANE ( 'NONE',  #16757 ) ;
#22580=EDGE_CURVE ( 'NONE', #25158, #2026, #12750, .T. ) ;
#22600=ORIENTED_EDGE ( 'NONE', *, *, #17453, .F. ) ;
#22608=CARTESIAN_POINT ( 'NONE',  ( 43.31606138205700063, -35.70002751211045933, 71.94742330197156832 ) ) ;
#22613=DIRECTION ( 'NONE',  ( 0.000000000000000000, 0.8212051873014208914, 0.5706330172266919076 ) ) ;
#22617=DIRECTION ( 'NONE',  ( 0.000000000000000000, -0.5706330172266920187, 0.8212051873014210024 ) ) ;
#22620=CARTESIAN_POINT ( 'NONE',  ( 43.23254934194437027, 3.260207155506757992, 6.242825920358057168 ) ) ;
#22623=DIRECTION ( 'NONE',  ( -1.849283715844614456E-16, 0.8212051873014208914, 0.5706330172266919076 ) ) ;
#22647=EDGE_CURVE ( 'NONE', #23614, #20521, #4222, .T. ) ;
#22650=CARTESIAN_POINT ( 'NONE',  ( 40.06606138205700063, 5.594015759443068170, 2.006005027196319901 ) ) ;
#22652=ORIENTED_EDGE ( 'NONE', *, *, #6983, .T. ) ;
#22664=ORIENTED_EDGE ( 'NONE', *, *, #10244, .F. ) ;
#22665=DIRECTION ( 'NONE',  ( 0.000000000000000000, -0.8212051873014223347, -0.5706330172266899092 ) ) ;
#22672=CARTESIAN_POINT ( 'NONE',  ( 42.56606138205700063, -33.77966242919868733, 58.66916295099436951 ) ) ;
#22695=AXIS2_PLACEMENT_3D ( 'NONE', #18836, #1176, #20902 ) ;
#22698=CYLINDRICAL_SURFACE ( 'NONE', #22695, 0.4999999999999998890 ) ;
#22705=VECTOR ( 'NONE', #14127, 1000.000000000000114 ) ;
#22713=EDGE_CURVE ( 'NONE', #14645, #3435, #10026, .T. ) ;
#22718=ORIENTED_EDGE ( 'NONE', *, *, #17453, .T. ) ;
#22727=CARTESIAN_POINT ( 'NONE',  ( 43.81606138205700063, 4.103895195095678794, 6.341006091748962348 ) ) ;
#22730=AXIS2_PLACEMENT_3D ( 'NONE', #15679, #21479, #1752 ) ;
#22731=CARTESIAN_POINT ( 'NONE',  ( 36.06606138205700063, 2.740850673309605412, 6.112030963703427133 ) ) ;
#22741=DIRECTION ( 'NONE',  ( -1.000000000000000000, 0.000000000000000000, 0.000000000000000000 ) ) ;
#22743=CARTESIAN_POINT ( 'NONE',  ( 42.99361969242278292, 2.839052459004266726, 6.102834979010582472 ) ) ;
#22746=VECTOR ( 'NONE', #23115, 1000.000000000000000 ) ;
#22768=DIRECTION ( 'NONE',  ( 1.000000000000000000, -0.000000000000000000, 0.000000000000000000 ) ) ;
#22769=CIRCLE ( 'NONE', #543, 0.4999999999999982792 ) ;
#22770=CARTESIAN_POINT ( 'NONE',  ( 40.56606138205700773, 2.740850673309605412, 6.112030963703427133 ) ) ;
#22781=DIRECTION ( 'NONE',  ( 1.000000000000000000, -0.000000000000000000, 0.000000000000000000 ) ) ;
#22784=EDGE_LOOP ( 'NONE', ( #16729, #15906, #8922, #23799 ) ) ;
#22818=VERTEX_POINT ( 'NONE', #12476 ) ;
#22840=DIRECTION ( 'NONE',  ( 1.445602896647340149E-16, -0.8212051873014210024, -0.5706330172266920187 ) ) ;
#22854=DIRECTION ( 'NONE',  ( 0.000000000000000000, -0.5706330172266915746, 0.8212051873014213355 ) ) ;
#22862=DIRECTION ( 'NONE',  ( -1.000000000000000000, 0.000000000000000000, 0.000000000000000000 ) ) ;
#22869=( NAMED_UNIT ( * ) PLANE_ANGLE_UNIT ( ) SI_UNIT ( $, .RADIAN. ) );
#22880=ORIENTED_EDGE ( 'NONE', *, *, #3075, .T. ) ;
#22899=VECTOR ( 'NONE', #21697, 1000.000000000000000 ) ;
#22904=ORIENTED_EDGE ( 'NONE', *, *, #2938, .F. ) ;
#22930=ORIENTED_EDGE ( 'NONE', *, *, #18309, .F. ) ;
#22960=CARTESIAN_POINT ( 'NONE',  ( 36.06606138205700063, 5.594015759443068170, 2.006005027196319901 ) ) ;
#22963=ADVANCED_FACE ( 'NONE', ( #19144 ), #13216, .T. ) ;
#22999=CIRCLE ( 'NONE', #14783, 0.4999999999999982792 ) ;
#23010=ORIENTED_EDGE ( 'NONE', *, *, #10782, .F. ) ;
#23018=CARTESIAN_POINT ( 'NONE',  ( 43.38751330861538236, 3.099072278389038981, 6.135933108610800879 ) ) ;
#23031=ORIENTED_EDGE ( 'NONE', *, *, #19250, .T. ) ;
#23035=CARTESIAN_POINT ( 'NONE',  ( 42.74055771317608787, 3.188265934946779012, 6.371314334530746137 ) ) ;
#23050=CIRCLE ( 'NONE', #9488, 2.500000000000002220 ) ;
#23063=CYLINDRICAL_SURFACE ( 'NONE', #11547, 2.500000000000002220 ) ;
#23078=CYLINDRICAL_SURFACE ( 'NONE', #11838, 0.4999999999999982792 ) ;
#23115=DIRECTION ( 'NONE',  ( -1.000000000000000000, 0.000000000000000000, 0.000000000000000000 ) ) ;
#23147=DIRECTION ( 'NONE',  ( -1.445602896647339656E-16, 0.8212051873014208914, 0.5706330172266919076 ) ) ;
#23149=DIRECTION ( 'NONE',  ( 0.000000000000000000, -0.5706330172266907974, 0.8212051873014217795 ) ) ;
#23170=CARTESIAN_POINT ( 'NONE',  ( 33.33121445922205339, -32.87633672316712108, 59.29685926994373091 ) ) ;
#23179=VERTEX_POINT ( 'NONE', #16025 ) ;
#23180=DIRECTION ( 'NONE',  ( -1.000000000000000000, 0.000000000000000000, 0.000000000000000000 ) ) ;
#23181=EDGE_CURVE ( 'NONE', #4360, #25460, #19328, .T. ) ;
#23201=CARTESIAN_POINT ( 'NONE',  ( 43.81606138205700063, -35.70002751211045933, 71.94742330197156832 ) ) ;
#23204=ORIENTED_EDGE ( 'NONE', *, *, #5793, .T. ) ;
#23237=EDGE_CURVE ( 'NONE', #13134, #25120, #6584, .T. ) ;
#23240=CARTESIAN_POINT ( 'NONE',  ( 43.31606138205700063, -37.98241563432385703, 69.85268917996594951 ) ) ;
#23242=SURFACE_SIDE_STYLE ('',( #15137 ) ) ;
#23245=CARTESIAN_POINT ( 'NONE',  ( 40.56606138205700773, 5.308699250829721272, 2.416607620847027960 ) ) ;
#23248=DIRECTION ( 'NONE',  ( -2.168404344971010101E-16, 0.8212051873014210024, 0.5706330172266920187 ) ) ;
#23274=CARTESIAN_POINT ( 'NONE',  ( 36.06606138205700063, 5.594015759443068170, 2.006005027196319901 ) ) ;
#23278=ADVANCED_FACE ( 'NONE', ( #10363 ), #18228, .F. ) ;
#23292=DIRECTION ( 'NONE',  ( -1.445602896647339656E-16, 0.8212051873014208914, 0.5706330172266919076 ) ) ;
#23301=CARTESIAN_POINT ( 'NONE',  ( 43.81606138205700063, -39.60075215179220720, 69.23691647014479145 ) ) ;
#23316=FACE_OUTER_BOUND ( 'NONE', #25066, .T. ) ;
#23317=VERTEX_POINT ( 'NONE', #22336 ) ;
#23331=CARTESIAN_POINT ( 'NONE',  ( 33.31606138205700773, 3.996716213179724697, 6.311483552851885115 ) ) ;
#23333=AXIS2_PLACEMENT_3D ( 'NONE', #12682, #801, #16918 ) ;
#23335=CARTESIAN_POINT ( 'NONE',  ( 34.06606138205700773, -36.11063010576116739, 71.66210679335823386 ) ) ;
#23369=CARTESIAN_POINT ( 'NONE',  ( 43.31097620601923381, -33.12114953149411178, 59.73560708446377987 ) ) ;
#23407=ORIENTED_EDGE ( 'NONE', *, *, #8159, .F. ) ;
#23423=ORIENTED_EDGE ( 'NONE', *, *, #839, .T. ) ;
#23424=AXIS2_PLACEMENT_3D ( 'NONE', #14014, #14142, #15813 ) ;
#23426=AXIS2_PLACEMENT_3D ( 'NONE', #14407, #4117, #12495 ) ;
#23430=VECTOR ( 'NONE', #2244, 1000.000000000000114 ) ;
#23432=EDGE_CURVE ( 'NONE', #21114, #2595, #18116, .T. ) ;
#23433=CARTESIAN_POINT ( 'NONE',  ( 43.06277394478077269, 3.412914273465426973, 6.350629194390777776 ) ) ;
#23439=CARTESIAN_POINT ( 'NONE',  ( 43.31606138205700063, -35.82531359714782582, 71.25150419970752580 ) ) ;
#23455=DIRECTION ( 'NONE',  ( 1.000000000000000000, -0.000000000000000000, 0.000000000000000000 ) ) ;
#23457=CARTESIAN_POINT ( 'NONE',  ( 33.91905694501954116, 2.753407105083469197, 6.093960844037363600 ) ) ;
#23478=ORIENTED_EDGE ( 'NONE', *, *, #8040, .T. ) ;
#23517=CARTESIAN_POINT ( 'NONE',  ( 42.56606138205700063, 2.740850673309605412, 6.112030963703427133 ) ) ;
#23532=VERTEX_POINT ( 'NONE', #15457 ) ;
#23533=ADVANCED_FACE ( 'NONE', ( #6057 ), #7478, .T. ) ;
#23534=VECTOR ( 'NONE', #24535, 1000.000000000000114 ) ;
#23548=VECTOR ( 'NONE', #14634, 1000.000000000000114 ) ;
#23558=LINE ( 'NONE', #12119, #22150 ) ;
#23560=CARTESIAN_POINT ( 'NONE',  ( 43.31606138205700063, -1.963190818658398173, 19.89143565483009013 ) ) ;
#23570=CIRCLE ( 'NONE', #8380, 0.5000000000000004441 ) ;
#23579=ORIENTED_EDGE ( 'NONE', *, *, #13196, .T. ) ;
#23591=EDGE_CURVE ( 'NONE', #5873, #19839, #17271, .T. ) ;
#23592=EDGE_CURVE ( 'NONE', #17862, #9175, #1657, .T. ) ;
#23603=DIRECTION ( 'NONE',  ( 0.000000000000000000, 0.5706330172266920187, -0.8212051873014210024 ) ) ;
#23610=VECTOR ( 'NONE', #14171, 1000.000000000000000 ) ;
#23614=VERTEX_POINT ( 'NONE', #13662 ) ;
#23620=ORIENTED_EDGE ( 'NONE', *, *, #8560, .T. ) ;
#23624=PLANE ( 'NONE',  #19519 ) ;
#23626=DIRECTION ( 'NONE',  ( -1.000000000000000000, -0.000000000000000000, 0.000000000000000000 ) ) ;
#23637=EDGE_LOOP ( 'NONE', ( #7312, #1005, #455, #20470 ) ) ;
#23666=DIRECTION ( 'NONE',  ( 0.000000000000000000, -0.8212051873014208914, -0.5706330172266919076 ) ) ;
#23683=CYLINDRICAL_SURFACE ( 'NONE', #10412, 0.4999999999999943379 ) ;
#23699=ORIENTED_EDGE ( 'NONE', *, *, #9784, .F. ) ;
#23705=CYLINDRICAL_SURFACE ( 'NONE', #16587, 1.250000000000001110 ) ;
#23717=LINE ( 'NONE', #6087, #14779 ) ;
#23729=CARTESIAN_POINT ( 'NONE',  ( 43.31606138205700063, -39.60075215179220720, 69.23691647014479145 ) ) ;
#23732=EDGE_CURVE ( 'NONE', #8708, #7878, #18168, .T. ) ;
#23779=ORIENTED_EDGE ( 'NONE', *, *, #20775, .F. ) ;
#23785=CARTESIAN_POINT ( 'NONE',  ( 33.57054761034910229, 3.412271088041349820, 6.349711998884802533 ) ) ;
#23791=ORIENTED_EDGE ( 'NONE', *, *, #12474, .T. ) ;
#23795=ORIENTED_EDGE ( 'NONE', *, *, #18408, .F. ) ;
#23799=ORIENTED_EDGE ( 'NONE', *, *, #9274, .F. ) ;
#23802=CARTESIAN_POINT ( 'NONE',  ( 43.27472635360392417, 2.989809604489832573, 6.109225132705429218 ) ) ;
#23807=ADVANCED_FACE ( 'NONE', ( #6438 ), #14178, .T. ) ;
#23817=ORIENTED_EDGE ( 'NONE', *, *, #16105, .T. ) ;
#23825=ORIENTED_EDGE ( 'NONE', *, *, #13592, .F. ) ;
#23838=PLANE ( 'NONE',  #10438 ) ;
#23871=EDGE_CURVE ( 'NONE', #22818, #2214, #23050, .T. ) ;
#23875=CARTESIAN_POINT ( 'NONE',  ( 42.56606138205700063, 3.151453266960317023, 6.397347472316774031 ) ) ;
#23877=DIRECTION ( 'NONE',  ( -1.000000000000000000, 0.000000000000000000, 0.000000000000000000 ) ) ;
#23881=EDGE_CURVE ( 'NONE', #4447, #8708, #17316, .T. ) ;
#23896=CARTESIAN_POINT ( 'NONE',  ( 32.81606138205700773, 2.761903742731119049, 12.21527246050395377 ) ) ;
#23900=ORIENTED_EDGE ( 'NONE', *, *, #19086, .F. ) ;
#23913=DIRECTION ( 'NONE',  ( 0.000000000000000000, -0.5706330172266839140, 0.8212051873014264425 ) ) ;
#23917=ORIENTED_EDGE ( 'NONE', *, *, #6981, .T. ) ;
#23928=FACE_OUTER_BOUND ( 'NONE', #7008, .T. ) ;
#23935=CARTESIAN_POINT ( 'NONE',  ( 43.06085842172421252, 3.410736059654636332, 6.350806888899277247 ) ) ;
#23984=FACE_OUTER_BOUND ( 'NONE', #20955, .T. ) ;
#23987=CARTESIAN_POINT ( 'NONE',  ( 43.31606138205700063, -25.26124097814961544, 70.06813202641110649 ) ) ;
#23991=EDGE_LOOP ( 'NONE', ( #5278, #9837, #17990, #20346 ) ) ;
#23992=CARTESIAN_POINT ( 'NONE',  ( 33.57054579126889138, 3.412273012123823168, 6.349712035633038987 ) ) ;
#24009=CARTESIAN_POINT ( 'NONE',  ( 36.06606138205700063, 2.740850673309605412, 6.112030963703427133 ) ) ;
#24026=VERTEX_POINT ( 'NONE', #13004 ) ;
#24043=EDGE_LOOP ( 'NONE', ( #24072, #5172, #9257, #24383 ) ) ;
#24045=DIRECTION ( 'NONE',  ( 0.000000000000000000, -0.5706330172266919076, 0.8212051873014208914 ) ) ;
#24057=LINE ( 'NONE', #4494, #9053 ) ;
#24058=DIRECTION ( 'NONE',  ( 1.000000000000000000, -0.000000000000000000, 0.000000000000000000 ) ) ;
#24072=ORIENTED_EDGE ( 'NONE', *, *, #3910, .F. ) ;
#24078=FACE_OUTER_BOUND ( 'NONE', #14107, .T. ) ;
#24108=CARTESIAN_POINT ( 'NONE',  ( 33.31606138205700773, 4.124002793203064066, 6.312068993173404863 ) ) ;
#24118=EDGE_LOOP ( 'NONE', ( #1372, #21060, #13041, #682, #12247, #21090, #22058, #9248, #12109 ) ) ;
#24132=ORIENTED_EDGE ( 'NONE', *, *, #21669, .T. ) ;
#24137=ORIENTED_EDGE ( 'NONE', *, *, #5400, .F. ) ;
#24141=VECTOR ( 'NONE', #12265, 1000.000000000000000 ) ;
#24148=CARTESIAN_POINT ( 'NONE',  ( 43.31606138205700063, -10.80800258567212602, 32.62011605800211811 ) ) ;
#24159=VERTEX_POINT ( 'NONE', #17371 ) ;
#24160=LINE ( 'NONE', #601, #2951 ) ;
#24163=ORIENTED_EDGE ( 'NONE', *, *, #9884, .T. ) ;
#24168=DIRECTION ( 'NONE',  ( 0.000000000000000000, 0.5706330172266920187, -0.8212051873014210024 ) ) ;
#24178=CARTESIAN_POINT ( 'NONE',  ( 43.52392165233022325, 3.236692751922551459, 6.150480132932879762 ) ) ;
#24180=EDGE_CURVE ( 'NONE', #4087, #6765, #4543, .T. ) ;
#24181=FACE_OUTER_BOUND ( 'NONE', #7948, .T. ) ;
#24192=CARTESIAN_POINT ( 'NONE',  ( 34.06606138205689405, 3.151453266960317023, 6.397347472316774031 ) ) ;
#24205=VECTOR ( 'NONE', #19113, 1000.000000000000000 ) ;
#24206=DIRECTION ( 'NONE',  ( 3.771137991253929559E-16, -0.8212051873014208914, -0.5706330172266919076 ) ) ;
#24208=AXIS2_PLACEMENT_3D ( 'NONE', #7993, #6432, #22136 ) ;
#24226=VERTEX_POINT ( 'NONE', #9775 ) ;
#24232=FACE_OUTER_BOUND ( 'NONE', #9550, .T. ) ;
#24246=CARTESIAN_POINT ( 'NONE',  ( 33.31606138205700773, -10.80800258567212602, 32.62011605800211811 ) ) ;
#24249=VECTOR ( 'NONE', #8658, 1000.000000000000000 ) ;
#24262=ORIENTED_EDGE ( 'NONE', *, *, #16831, .F. ) ;
#24269=ADVANCED_BREP_SHAPE_REPRESENTATION ( '', ( #16907, #2000 ), #17034 ) ;
#24307=VECTOR ( 'NONE', #14251, 1000.000000000000000 ) ;
#24309=ORIENTED_EDGE ( 'NONE', *, *, #25189, .T. ) ;
#24347=ORIENTED_EDGE ( 'NONE', *, *, #8023, .T. ) ;
#24351=LINE ( 'NONE', #2715, #20059 ) ;
#24367=LINE ( 'NONE', #12681, #12096 ) ;
#24372=PLANE ( 'NONE',  #19471 ) ;
#24373=DIRECTION ( 'NONE',  ( 0.000000000000000000, 0.8212051873014208914, 0.5706330172266919076 ) ) ;
#24383=ORIENTED_EDGE ( 'NONE', *, *, #8714, .F. ) ;
#24393=AXIS2_PLACEMENT_3D ( 'NONE', #16349, #2193, #14055 ) ;
#24407=AXIS2_PLACEMENT_3D ( 'NONE', #232, #6052, #4123 ) ;
#24417=VERTEX_POINT ( 'NONE', #10662 ) ;
#24418=EDGE_LOOP ( 'NONE', ( #11153, #12350, #14077, #16550 ) ) ;
#24435=DIRECTION ( 'NONE',  ( 0.000000000000000000, 0.8212051873014223347, 0.5706330172266899092 ) ) ;
#24456=CARTESIAN_POINT ( 'NONE',  ( 43.81606138205700063, -37.53049398575952722, 70.06662099985003067 ) ) ;
#24461=LINE ( 'NONE', #892, #24249 ) ;
#24513=VERTEX_POINT ( 'NONE', #20826 ) ;
#24527=CARTESIAN_POINT ( 'NONE',  ( 36.06606138205700063, 5.719301844480432884, 2.701924129460374413 ) ) ;
#24532=EDGE_LOOP ( 'NONE', ( #16656, #22664, #14639, #12994 ) ) ;
#24535=DIRECTION ( 'NONE',  ( 0.000000000000000000, -0.5706330172266919076, 0.8212051873014208914 ) ) ;
#24540=ORIENTED_EDGE ( 'NONE', *, *, #19347, .F. ) ;
#24541=VERTEX_POINT ( 'NONE', #9495 ) ;
#24555=CARTESIAN_POINT ( 'NONE',  ( 33.32114656318253054, -33.12114940777929917, 59.73560686274496589 ) ) ;
#24564=LINE ( 'NONE', #18421, #1648 ) ;
#24588=ORIENTED_EDGE ( 'NONE', *, *, #1683, .T. ) ;
#24593=CARTESIAN_POINT ( 'NONE',  ( 43.31606138205700063, -20.88462213363798270, 44.49284693533410717 ) ) ;
#24598=DIRECTION ( 'NONE',  ( -1.292986538149619279E-16, 0.9897030922575080769, 0.1431355622335914179 ) ) ;
#24601=CARTESIAN_POINT ( 'NONE',  ( 43.06468080341912241, 3.415100481987967562, 6.350457055188933886 ) ) ;
#24621=EDGE_CURVE ( 'NONE', #2595, #4447, #9626, .T. ) ;
#24624=LINE ( 'NONE', #10500, #1929 ) ;
#24627=ORIENTED_EDGE ( 'NONE', *, *, #21086, .T. ) ;
#24630=DIRECTION ( 'NONE',  ( 0.000000000000000000, -0.8212051873014223347, -0.5706330172266899092 ) ) ;
#24643=FACE_OUTER_BOUND ( 'NONE', #17743, .T. ) ;
#24653=CARTESIAN_POINT ( 'NONE',  ( 36.56606138205700063, 6.004618353093779781, 2.291321535809666354 ) ) ;
#24700=VECTOR ( 'NONE', #4445, 1000.000000000000114 ) ;
#24709=VERTEX_POINT ( 'NONE', #1861 ) ;
#24762=FACE_OUTER_BOUND ( 'NONE', #21596, .T. ) ;
#24765=VERTEX_POINT ( 'NONE', #8062 ) ;
#24775=CARTESIAN_POINT ( 'NONE',  ( 36.56606138205700063, 5.308699250829721272, 2.416607620847027960 ) ) ;
#24791=CARTESIAN_POINT ( 'NONE',  ( 35.81606138205700063, -6.959910619544162458, 20.07251914782757751 ) ) ;
#24812=PLANE ( 'NONE',  #19949 ) ;
#24816=CARTESIAN_POINT ( 'NONE',  ( 43.81606138205700063, -33.70281195181703993, 69.07320514641659770 ) ) ;
#24821=DIRECTION ( 'NONE',  ( 1.000000000000000000, 1.185526135920242153E-16, 8.246758300215675884E-17 ) ) ;
#24822=EDGE_CURVE ( 'NONE', #10938, #2026, #14238, .T. ) ;
#24823=EDGE_LOOP ( 'NONE', ( #5009, #2007, #1860, #494, #12333, #19273, #7415, #20733, #5082, #3044, #4240, #12972, #8889, #17795, #15836, #25007, #9046, #24627, #23779 ) ) ;
#24827=ORIENTED_EDGE ( 'NONE', *, *, #16616, .T. ) ;
#24844=PRODUCT_DEFINITION_FORMATION_WITH_SPECIFIED_SOURCE ( 'ANY', '', #10148, .NOT_KNOWN. ) ;
#24850=CARTESIAN_POINT ( 'NONE',  ( 33.31606138205700773, -37.81581049437288300, 70.47722359350072452 ) ) ;
#24862=CARTESIAN_POINT ( 'NONE',  ( 33.31606138205700773, -30.89740888249930961, 1.247106086993583718 ) ) ;
#24875=CYLINDRICAL_SURFACE ( 'NONE', #7990, 0.4999999999999982792 ) ;
#24887=CARTESIAN_POINT ( 'NONE',  ( 43.31606138205700063, -37.81581049437287589, 70.47722359350073873 ) ) ;
#24892=FACE_OUTER_BOUND ( 'NONE', #10971, .T. ) ;
#24916=DIRECTION ( 'NONE',  ( -1.000000000000000000, 0.000000000000000000, 0.000000000000000000 ) ) ;
#24925=CARTESIAN_POINT ( 'NONE',  ( 33.63430007298546087, 2.841684771932709186, 6.101742786271089791 ) ) ;
#24936=AXIS2_PLACEMENT_3D ( 'NONE', #4685, #12180, #10232 ) ;
#24972=CARTESIAN_POINT ( 'NONE',  ( 33.31606138205700773, -27.11289203277224402, 56.96090842897168471 ) ) ;
#24987=CARTESIAN_POINT ( 'NONE',  ( 43.81606138205700063, -40.21665604226827639, 68.80894170722476133 ) ) ;
#24995=ORIENTED_EDGE ( 'NONE', *, *, #15077, .T. ) ;
#25003=AXIS2_PLACEMENT_3D ( 'NONE', #8388, #5979, #19619 ) ;
#25007=ORIENTED_EDGE ( 'NONE', *, *, #10611, .T. ) ;
#25010=CARTESIAN_POINT ( 'NONE',  ( 33.56669025312701393, 3.416671603465565532, 6.349359658337636603 ) ) ;
#25018=CARTESIAN_POINT ( 'NONE',  ( 43.77584484464993153, 3.724255437227281362, 6.250601487277855028 ) ) ;
#25019=ORIENTED_EDGE ( 'NONE', *, *, #17138, .F. ) ;
#25022=VECTOR ( 'NONE', #20875, 1000.000000000000114 ) ;
#25024=CARTESIAN_POINT ( 'NONE',  ( 33.31606138205700773, -1.963190818658398173, 19.89143565483009013 ) ) ;
#25028=DIRECTION ( 'NONE',  ( 0.000000000000000000, 0.8212051873014208914, 0.5706330172266919076 ) ) ;
#25031=CARTESIAN_POINT ( 'NONE',  ( 43.31606138205700063, -33.60910547091194900, 60.61426200347987248 ) ) ;
#25033=CARTESIAN_POINT ( 'NONE',  ( 40.81606138205700773, -6.549308025893449070, 20.35783565644092619 ) ) ;
#25036=CIRCLE ( 'NONE', #6152, 0.4999999999999982792 ) ;
#25049=ORIENTED_EDGE ( 'NONE', *, *, #839, .F. ) ;
#25058=EDGE_CURVE ( 'NONE', #14856, #23614, #14852, .T. ) ;
#25066=EDGE_LOOP ( 'NONE', ( #1304, #25320, #7942, #21356 ) ) ;
#25078=CARTESIAN_POINT ( 'NONE',  ( 33.24019963865212191, 3.104051971978903701, 6.135536383744724098 ) ) ;
#25081=AXIS2_PLACEMENT_3D ( 'NONE', #20231, #2693, #6452 ) ;
#25087=VECTOR ( 'NONE', #14120, 1000.000000000000000 ) ;
#25094=DIRECTION ( 'NONE',  ( 0.000000000000000000, 0.5706330172266919076, -0.8212051873014208914 ) ) ;
#25095=DIRECTION ( 'NONE',  ( 1.000000000000000000, -0.000000000000000000, 0.000000000000000000 ) ) ;
#25120=VERTEX_POINT ( 'NONE', #22095 ) ;
#25124=CARTESIAN_POINT ( 'NONE',  ( 32.81606138205700773, 3.939299543010435389, 6.271589894995780234 ) ) ;
#25126=CYLINDRICAL_SURFACE ( 'NONE', #13530, 0.4999999999999998890 ) ;
#25128=EDGE_CURVE ( 'NONE', #6498, #24417, #10342, .T. ) ;
#25130=EDGE_CURVE ( 'NONE', #11454, #16162, #15915, .T. ) ;
#25137=DIRECTION ( 'NONE',  ( 0.000000000000000000, 0.1771812806364704007, 0.9841782327363373106 ) ) ;
#25145=ORIENTED_EDGE ( 'NONE', *, *, #22647, .T. ) ;
#25155=VECTOR ( 'NONE', #24045, 1000.000000000000114 ) ;
#25158=VERTEX_POINT ( 'NONE', #18123 ) ;
#25160=EDGE_CURVE ( 'NONE', #13577, #14856, #16166, .T. ) ;
#25176=FACE_OUTER_BOUND ( 'NONE', #2642, .T. ) ;
#25179=CARTESIAN_POINT ( 'NONE',  ( 42.85688703463539184, 2.786080299087619228, 6.091846835322635378 ) ) ;
#25180=AXIS2_PLACEMENT_3D ( 'NONE', #15828, #6045, #19826 ) ;
#25185=ORIENTED_EDGE ( 'NONE', *, *, #1683, .F. ) ;
#25187=PLANE ( 'NONE',  #15129 ) ;
#25189=EDGE_CURVE ( 'NONE', #11454, #4345, #9130, .T. ) ;
#25244=VERTEX_POINT ( 'NONE', #14867 ) ;
#25258=LINE ( 'NONE', #19224, #15764 ) ;
#25292=FACE_OUTER_BOUND ( 'NONE', #7023, .T. ) ;
#25298=DIRECTION ( 'NONE',  ( -1.000000000000000000, -1.187136597504755470E-16, -8.249087426255173666E-17 ) ) ;
#25301=EDGE_CURVE ( 'NONE', #22410, #8119, #17454, .T. ) ;
#25305=VECTOR ( 'NONE', #19184, 1000.000000000000000 ) ;
#25314=ORIENTED_EDGE ( 'NONE', *, *, #12112, .T. ) ;
#25320=ORIENTED_EDGE ( 'NONE', *, *, #3018, .T. ) ;
#25328=DIRECTION ( 'NONE',  ( 1.000000000000000000, -0.000000000000000000, 0.000000000000000000 ) ) ;
#25344=FACE_OUTER_BOUND ( 'NONE', #24532, .T. ) ;
#25375=LINE ( 'NONE', #21538, #15209 ) ;
#25377=CARTESIAN_POINT ( 'NONE',  ( 33.97785981918843845, 3.164009542231369654, 6.379277577875881455 ) ) ;
#25383=CARTESIAN_POINT ( 'NONE',  ( 33.42374909935192306, 3.629904212211158221, 6.320127632620215152 ) ) ;
#25393=VERTEX_POINT ( 'NONE', #20097 ) ;
#25405=VECTOR ( 'NONE', #833, 1000.000000000000114 ) ;
#25422=VECTOR ( 'NONE', #21106, 1000.000000000000227 ) ;
#25424=VERTEX_POINT ( 'NONE', #15634 ) ;
#25429=EDGE_CURVE ( 'NONE', #10938, #12466, #10649, .T. ) ;
#25435=LINE ( 'NONE', #16041, #11992 ) ;
#25459=DIRECTION ( 'NONE',  ( -1.000000000000000000, 0.000000000000000000, 0.000000000000000000 ) ) ;
#25460=VERTEX_POINT ( 'NONE', #14304 ) ;
#25485=CARTESIAN_POINT ( 'NONE',  ( 43.06468080341912241, 3.415100481987967562, 6.350457055188933886 ) ) ;
#25486=VECTOR ( 'NONE', #18639, 1000.000000000000114 ) ;
ENDSEC;
END-ISO-10303-21;
